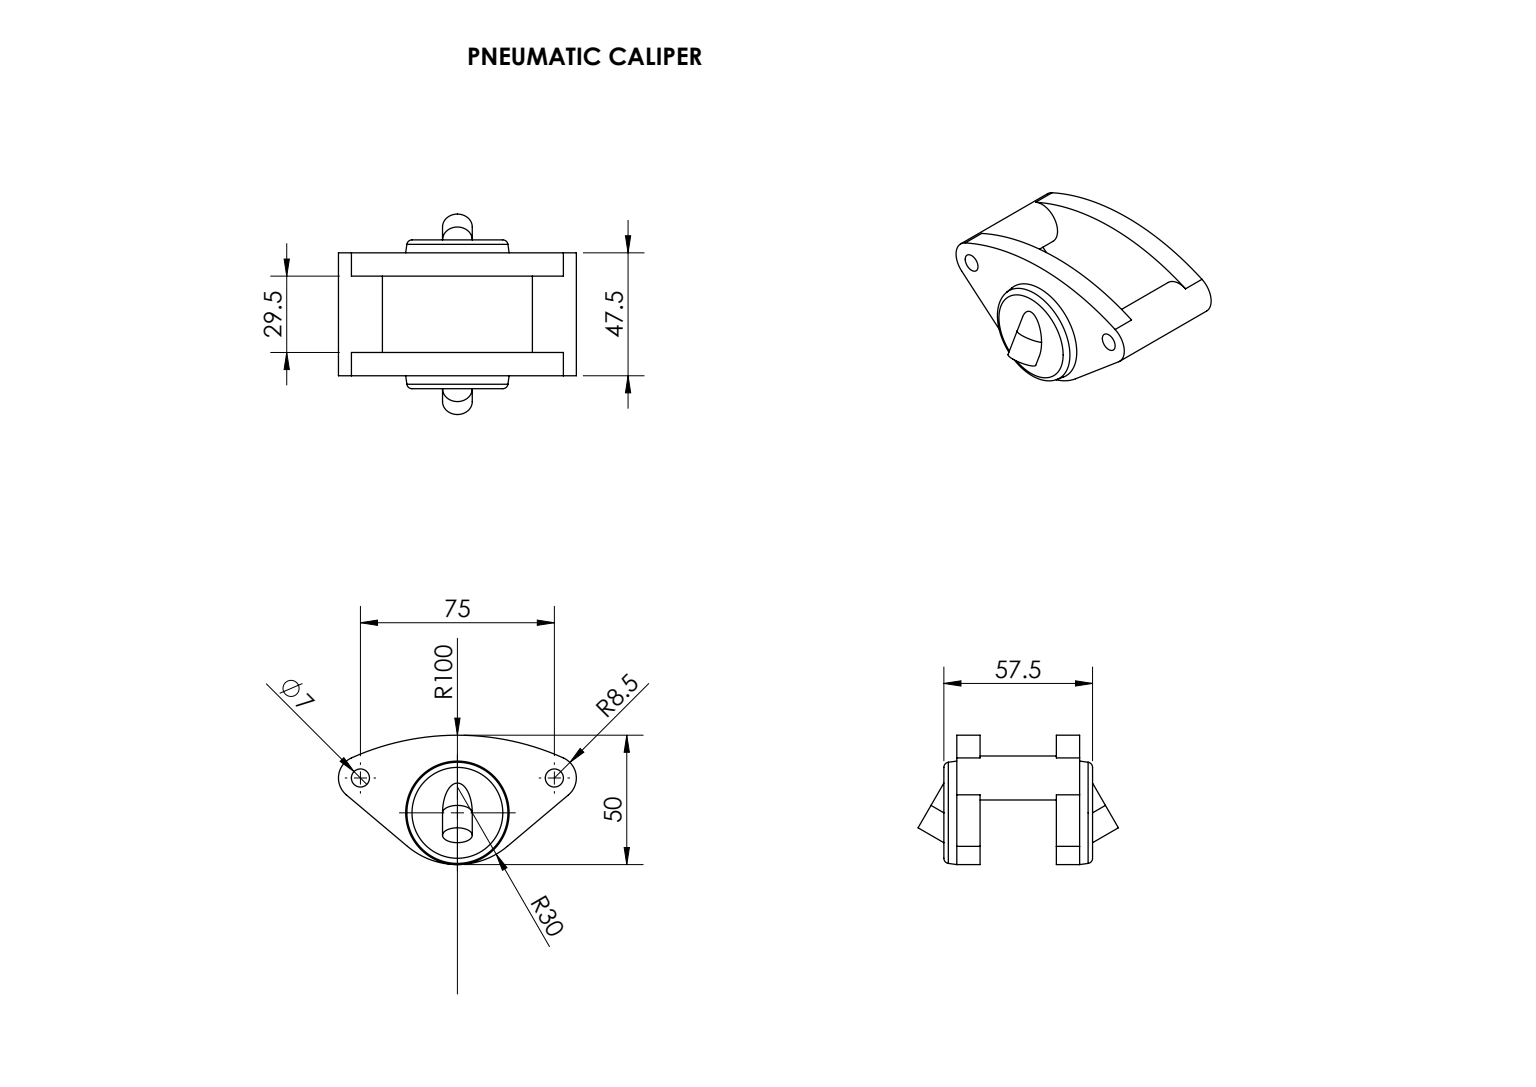
ISO-10303-21;
HEADER;
FILE_DESCRIPTION (('STEP AP214'),
    '1' );
FILE_NAME ('Pneumatic caliper.step',
    '2026-09-21T15:58:29',
    ( '' ),
    ( '' ),
    'SwSTEP 2.0',
    'SolidWorks 2026',
    '' );
FILE_SCHEMA (( 'AUTOMOTIVE_DESIGN' ));
ENDSEC;

DATA;
#6=AXIS2_PLACEMENT_3D ( 'NONE', #11763, #3538, #9529 ) ;
#8=ADVANCED_FACE ( 'NONE', ( #25357 ), #3421, .T. ) ;
#26=DIRECTION ( 'NONE',  ( 0.000000000000000000, 0.4999999999999951150, -0.8660254037844414832 ) ) ;
#43=LINE ( 'NONE', #5489, #22981 ) ;
#65=LINE ( 'NONE', #14323, #21127 ) ;
#74=CARTESIAN_POINT ( 'NONE',  ( -5.750000000000000000, 96.68456697298042002, 32.49999999999999289 ) ) ;
#105=VERTEX_POINT ( 'NONE', #9030 ) ;
#134=ORIENTED_EDGE ( 'NONE', *, *, #2252, .T. ) ;
#160=PRODUCT ( 'Pneumatic caliper', 'Pneumatic caliper', '', ( #18111 ) ) ;
#162=CARTESIAN_POINT ( 'NONE',  ( -2.448772250512182280E-15, 99.94802294027086020, -19.99999999999999645 ) ) ;
#175=CARTESIAN_POINT ( 'NONE',  ( -37.50000000000000000, 103.4105893997321886, -19.99999999999999645 ) ) ;
#283=ORIENTED_EDGE ( 'NONE', *, *, #11463, .F. ) ;
#335=ORIENTED_EDGE ( 'NONE', *, *, #20881, .T. ) ;
#374=VERTEX_POINT ( 'NONE', #8609 ) ;
#431=DIRECTION ( 'NONE',  ( 1.000000000000000000, 0.000000000000000000, 0.000000000000000000 ) ) ;
#441=ORIENTED_EDGE ( 'NONE', *, *, #21012, .F. ) ;
#469=EDGE_CURVE ( 'NONE', #105, #36472, #11048, .T. ) ;
#493=EDGE_CURVE ( 'NONE', #20027, #19694, #7016, .T. ) ;
#530=VERTEX_POINT ( 'NONE', #7444 ) ;
#537=CARTESIAN_POINT ( 'NONE',  ( -37.50000000000000000, 103.4105893997321886, 27.49999999999999645 ) ) ;
#544=CARTESIAN_POINT ( 'NONE',  ( 40.98360655737705116, 111.1639425680974398, -19.99999999999999645 ) ) ;
#554=EDGE_CURVE ( 'NONE', #14180, #7296, #6835, .T. ) ;
#576=CARTESIAN_POINT ( 'NONE',  ( 3.368272016354729725, 78.44802294027070388, 32.49999999999999289 ) ) ;
#585=DIRECTION ( 'NONE',  ( 0.000000000000000000, -0.000000000000000000, 1.000000000000000000 ) ) ;
#623=VERTEX_POINT ( 'NONE', #30682 ) ;
#651=DIRECTION ( 'NONE',  ( 1.000000000000000000, 0.000000000000000000, 0.000000000000000000 ) ) ;
#681=EDGE_CURVE ( 'NONE', #4131, #30183, #32146, .T. ) ;
#692=CYLINDRICAL_SURFACE ( 'NONE', #6427, 5.750000000000005329 ) ;
#705=FACE_OUTER_BOUND ( 'NONE', #31997, .T. ) ;
#721=CARTESIAN_POINT ( 'NONE',  ( 40.98360655737705116, 111.1639425680974398, 27.49999999999999645 ) ) ;
#750=CARTESIAN_POINT ( 'NONE',  ( -7.041719095097282852E-16, 78.44802294027068967, 32.49999999999999289 ) ) ;
#755=VERTEX_POINT ( 'NONE', #25262 ) ;
#856=CARTESIAN_POINT ( 'NONE',  ( 19.31922176934805435, 76.99660315353983719, -11.00000000000000000 ) ) ;
#927=CARTESIAN_POINT ( 'NONE',  ( 46.00000000000000000, 103.4105893997321743, -19.99999999999999645 ) ) ;
#950=EDGE_CURVE ( 'NONE', #15883, #26378, #23725, .T. ) ;
#958=VECTOR ( 'NONE', #35917, 1000.000000000000000 ) ;
#983=AXIS2_PLACEMENT_3D ( 'NONE', #1559, #4573, #18819 ) ;
#1027=CARTESIAN_POINT ( 'NONE',  ( -33.99999999999999289, 103.4105893997321886, -19.99999999999999645 ) ) ;
#1082=CARTESIAN_POINT ( 'NONE',  ( 37.50000000000000000, 103.4105893997321743, -19.99999999999999645 ) ) ;
#1097=DIRECTION ( 'NONE',  ( 0.000000000000000000, -0.8660254037844420383, -0.4999999999999945599 ) ) ;
#1190=ORIENTED_EDGE ( 'NONE', *, *, #24796, .T. ) ;
#1228=ORIENTED_EDGE ( 'NONE', *, *, #33762, .F. ) ;
#1243=DIRECTION ( 'NONE',  ( -0.000000000000000000, -0.000000000000000000, 1.000000000000000000 ) ) ;
#1432=ORIENTED_EDGE ( 'NONE', *, *, #33576, .T. ) ;
#1488=CIRCLE ( 'NONE', #28409, 1.750000000000018652 ) ;
#1509=ORIENTED_EDGE ( 'NONE', *, *, #29374, .F. ) ;
#1513=DIRECTION ( 'NONE',  ( 0.000000000000000000, 0.4999999999999953926, 0.8660254037844412611 ) ) ;
#1518=DIRECTION ( 'NONE',  ( -0.000000000000000000, -0.000000000000000000, 1.000000000000000000 ) ) ;
#1531=ORIENTED_EDGE ( 'NONE', *, *, #950, .F. ) ;
#1540=AXIS2_PLACEMENT_3D ( 'NONE', #7269, #15702, #21694 ) ;
#1559=CARTESIAN_POINT ( 'NONE',  ( 0.000000000000000000, 89.94802294027088863, 27.49999999999999645 ) ) ;
#1579=CARTESIAN_POINT ( 'NONE',  ( 42.97377950131527058, 96.90768712682506703, -19.99999999999999645 ) ) ;
#1619=DIRECTION ( 'NONE',  ( 0.000000000000000000, -0.000000000000000000, 1.000000000000000000 ) ) ;
#1622=EDGE_CURVE ( 'NONE', #20027, #10852, #65, .T. ) ;
#1690=LINE ( 'NONE', #32433, #24985 ) ;
#1707=DIRECTION ( 'NONE',  ( 0.000000000000000000, 0.000000000000000000, 1.000000000000000000 ) ) ;
#1771=CARTESIAN_POINT ( 'NONE',  ( 0.000000000000000000, 84.16276890242652087, 42.47964607176039209 ) ) ;
#1854=ADVANCED_BREP_SHAPE_REPRESENTATION ( '', ( #32508, #21385 ), #29775 ) ;
#1871=PLANE ( 'NONE',  #17245 ) ;
#1872=ORIENTED_EDGE ( 'NONE', *, *, #18822, .T. ) ;
#1907=FACE_BOUND ( 'NONE', #19435, .T. ) ;
#1911=CARTESIAN_POINT ( 'NONE',  ( 0.000000000000000000, 81.28776890242656350, 37.49999999999985079 ) ) ;
#1925=EDGE_LOOP ( 'NONE', ( #10034, #14549, #26368, #1432 ) ) ;
#1928=CARTESIAN_POINT ( 'NONE',  ( 19.31922176934805435, 76.99660315353983719, 18.49999999999999645 ) ) ;
#1999=CARTESIAN_POINT ( 'NONE',  ( 5.750000000000000000, 89.94802294027094547, -24.99999999999999645 ) ) ;
#2018=DIRECTION ( 'NONE',  ( 0.000000000000000000, -0.8660254037844420383, -0.4999999999999945599 ) ) ;
#2092=ADVANCED_FACE ( 'NONE', ( #33123 ), #7443, .F. ) ;
#2180=CARTESIAN_POINT ( 'NONE',  ( -2.775557561562891351E-14, 19.94802294027085310, 27.49999999999999645 ) ) ;
#2187=DIRECTION ( 'NONE',  ( -1.000000000000000000, 0.000000000000000000, 0.000000000000000000 ) ) ;
#2193=CARTESIAN_POINT ( 'NONE',  ( -3.368272016354703968, 101.4480229402710592, 32.49999999999999289 ) ) ;
#2207=ADVANCED_FACE ( 'NONE', ( #24326 ), #10261, .F. ) ;
#2222=AXIS2_PLACEMENT_3D ( 'NONE', #29319, #32113, #20494 ) ;
#2228=ORIENTED_EDGE ( 'NONE', *, *, #950, .T. ) ;
#2252=EDGE_CURVE ( 'NONE', #24938, #36272, #5855, .T. ) ;
#2262=DIRECTION ( 'NONE',  ( -1.000000000000000000, 0.000000000000000000, 0.000000000000000000 ) ) ;
#2268=AXIS2_PLACEMENT_3D ( 'NONE', #6413, #29284, #22929 ) ;
#2294=EDGE_CURVE ( 'NONE', #12700, #36472, #17833, .T. ) ;
#2349=EDGE_CURVE ( 'NONE', #5579, #28337, #19633, .T. ) ;
#2398=AXIS2_PLACEMENT_3D ( 'NONE', #17153, #19603, #14518 ) ;
#2405=AXIS2_PLACEMENT_3D ( 'NONE', #24464, #16022, #21641 ) ;
#2437=FACE_BOUND ( 'NONE', #33052, .T. ) ;
#2439=CYLINDRICAL_SURFACE ( 'NONE', #3558, 5.750000000000002665 ) ;
#2454=CARTESIAN_POINT ( 'NONE',  ( -7.041719095097282852E-16, 87.07302294027100231, 27.52035392823936633 ) ) ;
#2478=DIRECTION ( 'NONE',  ( -0.000000000000000000, -0.000000000000000000, 1.000000000000000000 ) ) ;
#2492=DIRECTION ( 'NONE',  ( -0.000000000000000000, 0.8660254037844420383, -0.4999999999999945599 ) ) ;
#2516=LINE ( 'NONE', #31197, #12942 ) ;
#2582=CYLINDRICAL_SURFACE ( 'NONE', #11940, 8.500000000000003553 ) ;
#2620=CARTESIAN_POINT ( 'NONE',  ( 0.000000000000000000, 89.94802294027088863, 30.77834620192012594 ) ) ;
#2678=DIRECTION ( 'NONE',  ( 0.000000000000000000, 0.000000000000000000, -1.000000000000000000 ) ) ;
#2688=DIRECTION ( 'NONE',  ( -0.000000000000000000, -0.000000000000000000, -1.000000000000000000 ) ) ;
#2707=AXIS2_PLACEMENT_3D ( 'NONE', #5216, #2018, #20008 ) ;
#2814=ORIENTED_EDGE ( 'NONE', *, *, #21581, .T. ) ;
#2937=ORIENTED_EDGE ( 'NONE', *, *, #18375, .T. ) ;
#2945=EDGE_CURVE ( 'NONE', #374, #33065, #32532, .T. ) ;
#2967=DIRECTION ( 'NONE',  ( 0.000000000000000000, 0.000000000000000000, -1.000000000000000000 ) ) ;
#3005=SURFACE_STYLE_USAGE ( .BOTH. , #36939 ) ;
#3025=DIRECTION ( 'NONE',  ( 0.000000000000000000, -0.8660254037844419273, 0.4999999999999945599 ) ) ;
#3049=FACE_BOUND ( 'NONE', #20436, .T. ) ;
#3106=DIRECTION ( 'NONE',  ( -1.000000000000000000, 0.000000000000000000, 0.000000000000000000 ) ) ;
#3130=CARTESIAN_POINT ( 'NONE',  ( 0.000000000000000000, 81.28776890242656350, -29.99999999999985434 ) ) ;
#3139=CARTESIAN_POINT ( 'NONE',  ( 0.000000000000000000, 89.94802294027097389, -24.99999999999990763 ) ) ;
#3154=EDGE_LOOP ( 'NONE', ( #27426, #3715 ) ) ;
#3161=CARTESIAN_POINT ( 'NONE',  ( 0.000000000000000000, 89.94802294027088863, -24.99999999999999645 ) ) ;
#3167=VERTEX_POINT ( 'NONE', #4549 ) ;
#3178=ORIENTED_EDGE ( 'NONE', *, *, #493, .T. ) ;
#3242=LINE ( 'NONE', #17667, #10545 ) ;
#3254=VERTEX_POINT ( 'NONE', #22529 ) ;
#3267=DIRECTION ( 'NONE',  ( 1.000000000000000000, 0.000000000000000000, 0.000000000000000000 ) ) ;
#3338=ORIENTED_EDGE ( 'NONE', *, *, #7196, .T. ) ;
#3362=VECTOR ( 'NONE', #20623, 1000.000000000000000 ) ;
#3404=ORIENTED_EDGE ( 'NONE', *, *, #19687, .T. ) ;
#3411=DIRECTION ( 'NONE',  ( 0.000000000000000000, -1.000000000000000000, 0.000000000000000000 ) ) ;
#3415=AXIS2_PLACEMENT_3D ( 'NONE', #24206, #30396, #7341 ) ;
#3421=TOROIDAL_SURFACE ( 'NONE', #24386, 17.55872235085560007, 2.000000000000000000 ) ;
#3425=CARTESIAN_POINT ( 'NONE',  ( 37.50000000000000000, 103.4105893997321743, -19.99999999999999645 ) ) ;
#3432=VERTEX_POINT ( 'NONE', #34894 ) ;
#3476=AXIS2_PLACEMENT_3D ( 'NONE', #10985, #5195, #16826 ) ;
#3492=ORIENTED_EDGE ( 'NONE', *, *, #17442, .F. ) ;
#3538=DIRECTION ( 'NONE',  ( -0.000000000000000000, -0.000000000000000000, 1.000000000000000000 ) ) ;
#3550=ORIENTED_EDGE ( 'NONE', *, *, #19687, .F. ) ;
#3558=AXIS2_PLACEMENT_3D ( 'NONE', #31282, #17035, #28469 ) ;
#3585=CARTESIAN_POINT ( 'NONE',  ( 5.750000000000035527, 83.21147890756138565, 32.49999999999999289 ) ) ;
#3645=LINE ( 'NONE', #15074, #20651 ) ;
#3651=CARTESIAN_POINT ( 'NONE',  ( -28.99999999999998934, 103.4105893997321886, -11.00000000000000355 ) ) ;
#3715=ORIENTED_EDGE ( 'NONE', *, *, #27481, .F. ) ;
#3739=DIRECTION ( 'NONE',  ( 1.000000000000000000, 0.000000000000000000, 0.000000000000000000 ) ) ;
#3743=FACE_OUTER_BOUND ( 'NONE', #7188, .T. ) ;
#3776=DIRECTION ( 'NONE',  ( -0.000000000000000000, -0.000000000000000000, 1.000000000000000000 ) ) ;
#3779=DIRECTION ( 'NONE',  ( 0.000000000000000000, 0.000000000000000000, -1.000000000000000000 ) ) ;
#3785=DIRECTION ( 'NONE',  ( -1.000000000000000000, 0.000000000000000000, 0.000000000000000000 ) ) ;
#3796=ORIENTED_EDGE ( 'NONE', *, *, #31417, .F. ) ;
#3819=ADVANCED_FACE ( 'NONE', ( #28664 ), #2439, .T. ) ;
#3840=DIRECTION ( 'NONE',  ( -0.000000000000000000, -0.000000000000000000, -1.000000000000000000 ) ) ;
#3868=CARTESIAN_POINT ( 'NONE',  ( 0.000000000000000000, 98.60827697811544112, -19.99999999999999645 ) ) ;
#3871=VECTOR ( 'NONE', #23270, 1000.000000000000000 ) ;
#3883=DIRECTION ( 'NONE',  ( 0.6439740589782694258, 0.7650473262243666639, 0.000000000000000000 ) ) ;
#3895=CIRCLE ( 'NONE', #24270, 17.55872235085560007 ) ;
#3909=ORIENTED_EDGE ( 'NONE', *, *, #33038, .T. ) ;
#3956=VECTOR ( 'NONE', #20517, 1000.000000000000000 ) ;
#3970=LINE ( 'NONE', #6607, #19644 ) ;
#3978=CARTESIAN_POINT ( 'NONE',  ( 37.50000000000000000, 103.4105893997321743, -11.00000000000000355 ) ) ;
#3980=CARTESIAN_POINT ( 'NONE',  ( -42.97377950131527058, 96.90768712682508124, 18.49999999999999645 ) ) ;
#4025=CARTESIAN_POINT ( 'NONE',  ( -28.99999999999998934, 103.4105893997321886, 18.49999999999999645 ) ) ;
#4050=VERTEX_POINT ( 'NONE', #5357 ) ;
#4058=EDGE_CURVE ( 'NONE', #16958, #13946, #30472, .T. ) ;
#4094=FILL_AREA_STYLE_COLOUR ( '', #11095 ) ;
#4096=AXIS2_PLACEMENT_3D ( 'NONE', #31153, #25722, #11273 ) ;
#4099=DIRECTION ( 'NONE',  ( -0.000000000000000000, -0.000000000000000000, -1.000000000000000000 ) ) ;
#4131=VERTEX_POINT ( 'NONE', #30645 ) ;
#4151=CARTESIAN_POINT ( 'NONE',  ( 19.31922176934805435, 76.99660315353983719, -19.99999999999999645 ) ) ;
#4153=VECTOR ( 'NONE', #5154, 1000.000000000000000 ) ;
#4164=ORIENTED_EDGE ( 'NONE', *, *, #15491, .F. ) ;
#4167=ORIENTED_EDGE ( 'NONE', *, *, #23423, .F. ) ;
#4229=DIRECTION ( 'NONE',  ( -0.000000000000000000, -0.000000000000000000, -1.000000000000000000 ) ) ;
#4230=ORIENTED_EDGE ( 'NONE', *, *, #10722, .F. ) ;
#4234=EDGE_LOOP ( 'NONE', ( #22115, #32877 ) ) ;
#4257=CARTESIAN_POINT ( 'NONE',  ( 0.000000000000000000, 85.61789592134881843, -27.49999999999990408 ) ) ;
#4343=CARTESIAN_POINT ( 'NONE',  ( 0.000000000000000000, 98.60827697811544112, 27.49999999999999645 ) ) ;
#4363=ORIENTED_EDGE ( 'NONE', *, *, #23423, .T. ) ;
#4408=AXIS2_PLACEMENT_3D ( 'NONE', #21823, #33261, #16774 ) ;
#4410=CARTESIAN_POINT ( 'NONE',  ( 37.50000000000000000, 103.4105893997321743, 27.49999999999999645 ) ) ;
#4445=AXIS2_PLACEMENT_3D ( 'NONE', #30967, #8096, #25528 ) ;
#4450=DIRECTION ( 'NONE',  ( -0.000000000000000000, -0.000000000000000000, -1.000000000000000000 ) ) ;
#4475=ORIENTED_EDGE ( 'NONE', *, *, #30097, .T. ) ;
#4479=VECTOR ( 'NONE', #26592, 1000.000000000000000 ) ;
#4530=DIRECTION ( 'NONE',  ( -0.000000000000000000, -0.8660254037844414832, 0.4999999999999953371 ) ) ;
#4549=CARTESIAN_POINT ( 'NONE',  ( 7.041719095097282852E-16, 78.41276890242659192, -25.02035392823930593 ) ) ;
#4556=VERTEX_POINT ( 'NONE', #4560 ) ;
#4560=CARTESIAN_POINT ( 'NONE',  ( -7.041719095097282852E-16, 78.44802294027068967, 32.49999999999999289 ) ) ;
#4571=ORIENTED_EDGE ( 'NONE', *, *, #11658, .F. ) ;
#4573=DIRECTION ( 'NONE',  ( 0.000000000000000000, 0.000000000000000000, -1.000000000000000000 ) ) ;
#4580=FACE_BOUND ( 'NONE', #4234, .T. ) ;
#4585=LINE ( 'NONE', #24827, #34492 ) ;
#4596=EDGE_CURVE ( 'NONE', #34855, #18201, #32666, .T. ) ;
#4610=VERTEX_POINT ( 'NONE', #20447 ) ;
#4626=ADVANCED_FACE ( 'NONE', ( #28524, #28718, #3049 ), #28332, .F. ) ;
#4627=CARTESIAN_POINT ( 'NONE',  ( 0.000000000000000000, 82.16276890242660613, -31.51554445662266346 ) ) ;
#4633=CARTESIAN_POINT ( 'NONE',  ( 0.000000000000000000, 81.28776890242660613, -29.99999999999987566 ) ) ;
#4651=ORIENTED_EDGE ( 'NONE', *, *, #21027, .F. ) ;
#4666=CIRCLE ( 'NONE', #24411, 20.00000000000001066 ) ;
#4734=ORIENTED_EDGE ( 'NONE', *, *, #30255, .T. ) ;
#4760=VERTEX_POINT ( 'NONE', #35081 ) ;
#4769=AXIS2_PLACEMENT_3D ( 'NONE', #27991, #7760, #16371 ) ;
#4812=ORIENTED_EDGE ( 'NONE', *, *, #35492, .T. ) ;
#4827=EDGE_CURVE ( 'NONE', #22247, #15238, #15196, .T. ) ;
#4922=ORIENTED_EDGE ( 'NONE', *, *, #23505, .T. ) ;
#4934=DIRECTION ( 'NONE',  ( 0.000000000000000000, -0.8660254037844419273, 0.4999999999999945044 ) ) ;
#4964=CARTESIAN_POINT ( 'NONE',  ( 0.000000000000000000, 89.94802294027088863, 27.49999999999999645 ) ) ;
#5066=CARTESIAN_POINT ( 'NONE',  ( -41.00000000000000000, 103.4105893997321886, -19.99999999999999645 ) ) ;
#5149=ORIENTED_EDGE ( 'NONE', *, *, #31933, .T. ) ;
#5154=DIRECTION ( 'NONE',  ( -0.7650473262243666639, 0.6439740589782693148, -0.000000000000000000 ) ) ;
#5164=VECTOR ( 'NONE', #15215, 1000.000000000000114 ) ;
#5181=ADVANCED_FACE ( 'NONE', ( #32325 ), #28520, .T. ) ;
#5195=DIRECTION ( 'NONE',  ( -0.000000000000000000, -0.000000000000000000, -1.000000000000000000 ) ) ;
#5206=CARTESIAN_POINT ( 'NONE',  ( 0.000000000000000000, 101.4480229402710592, -24.99999999999999645 ) ) ;
#5216=CARTESIAN_POINT ( 'NONE',  ( 0.000000000000000000, 81.28776890242656350, -29.99999999999985434 ) ) ;
#5217=AXIS2_PLACEMENT_3D ( 'NONE', #21560, #24571, #32991 ) ;
#5218=FACE_OUTER_BOUND ( 'NONE', #16123, .T. ) ;
#5245=CIRCLE ( 'NONE', #6439, 8.500000000000000000 ) ;
#5256=STYLED_ITEM ( 'NONE', ( #28128 ), #1854 ) ;
#5266=FILL_AREA_STYLE ('',( #5811 ) ) ;
#5300=CIRCLE ( 'NONE', #30417, 2.000000000000001776 ) ;
#5329=ORIENTED_EDGE ( 'NONE', *, *, #24410, .F. ) ;
#5357=CARTESIAN_POINT ( 'NONE',  ( 40.98360655737705827, 111.1639425680974540, -11.00000000000000355 ) ) ;
#5428=CARTESIAN_POINT ( 'NONE',  ( 0.000000000000000000, 89.94802294027088863, 27.49999999999999645 ) ) ;
#5448=ADVANCED_FACE ( 'NONE', ( #20294 ), #31526, .F. ) ;
#5489=CARTESIAN_POINT ( 'NONE',  ( 0.000000000000000000, 86.49289592134881843, -29.01554445662268833 ) ) ;
#5512=CARTESIAN_POINT ( 'NONE',  ( 42.97377950131527058, 96.90768712682506703, -11.00000000000000000 ) ) ;
#5577=CARTESIAN_POINT ( 'NONE',  ( 0.000000000000000000, 89.94802294027094547, 32.49999999999999289 ) ) ;
#5579=VERTEX_POINT ( 'NONE', #13277 ) ;
#5591=FACE_OUTER_BOUND ( 'NONE', #29113, .T. ) ;
#5613=( NAMED_UNIT ( * ) PLANE_ANGLE_UNIT ( ) SI_UNIT ( $, .RADIAN. ) );
#5627=DIRECTION ( 'NONE',  ( 0.000000000000000000, -0.8660254037844419273, -0.4999999999999945599 ) ) ;
#5649=CIRCLE ( 'NONE', #35593, 19.53925848833874213 ) ;
#5652=VECTOR ( 'NONE', #24376, 1000.000000000000000 ) ;
#5665=CARTESIAN_POINT ( 'NONE',  ( 0.000000000000000000, 81.28776890242656350, 37.49999999999985079 ) ) ;
#5710=AXIS2_PLACEMENT_3D ( 'NONE', #29491, #23899, #34952 ) ;
#5712=CYLINDRICAL_SURFACE ( 'NONE', #27964, 5.750000000000002665 ) ;
#5755=CIRCLE ( 'NONE', #10513, 8.500000000000003553 ) ;
#5768=DIRECTION ( 'NONE',  ( -0.000000000000000000, -0.000000000000000000, 1.000000000000000000 ) ) ;
#5782=CIRCLE ( 'NONE', #10573, 5.750000000000005329 ) ;
#5811=FILL_AREA_STYLE_COLOUR ( '', #29097 ) ;
#5832=CARTESIAN_POINT ( 'NONE',  ( -2.775557561562891351E-14, 19.94802294027085310, 18.49999999999999645 ) ) ;
#5849=ORIENTED_EDGE ( 'NONE', *, *, #21287, .T. ) ;
#5852=CARTESIAN_POINT ( 'NONE',  ( 41.00000000000000000, 103.4105893997321743, -19.99999999999999645 ) ) ;
#5853=DIRECTION ( 'NONE',  ( 1.000000000000000000, 0.000000000000000000, 0.000000000000000000 ) ) ;
#5855=CIRCLE ( 'NONE', #8268, 1.750000000000015765 ) ;
#5892=VECTOR ( 'NONE', #6515, 999.9999999999998863 ) ;
#5900=ORIENTED_EDGE ( 'NONE', *, *, #31535, .F. ) ;
#5904=ADVANCED_FACE ( 'NONE', ( #31800 ), #692, .T. ) ;
#5941=EDGE_LOOP ( 'NONE', ( #16432, #3338, #5149, #21200 ) ) ;
#5956=DIRECTION ( 'NONE',  ( -0.000000000000000000, 0.000000000000000000, -1.000000000000000000 ) ) ;
#5970=CYLINDRICAL_SURFACE ( 'NONE', #29208, 5.750000000000002665 ) ;
#5977=AXIS2_PLACEMENT_3D ( 'NONE', #8755, #5956, #17387 ) ;
#6063=CARTESIAN_POINT ( 'NONE',  ( -2.448772250512182280E-15, 99.94802294027086020, 18.49999999999999645 ) ) ;
#6143=DIRECTION ( 'NONE',  ( -1.000000000000000000, 1.632680918566405215E-15, 0.000000000000000000 ) ) ;
#6151=EDGE_CURVE ( 'NONE', #16958, #30923, #25075, .T. ) ;
#6179=LINE ( 'NONE', #8815, #21940 ) ;
#6216=LINE ( 'NONE', #17648, #15504 ) ;
#6225=AXIS2_PLACEMENT_3D ( 'NONE', #4410, #3840, #29708 ) ;
#6236=ORIENTED_EDGE ( 'NONE', *, *, #10351, .T. ) ;
#6252=VERTEX_POINT ( 'NONE', #22808 ) ;
#6253=VERTEX_POINT ( 'NONE', #8543 ) ;
#6258=ORIENTED_EDGE ( 'NONE', *, *, #31855, .F. ) ;
#6299=DIRECTION ( 'NONE',  ( 0.000000000000000000, -0.8660254037844420383, -0.4999999999999945599 ) ) ;
#6312=DIRECTION ( 'NONE',  ( 0.000000000000000000, 0.4999999999999953926, -0.8660254037844412611 ) ) ;
#6384=CARTESIAN_POINT ( 'NONE',  ( -5.750000000000000000, 89.94802294027094547, -24.99999999999999645 ) ) ;
#6413=CARTESIAN_POINT ( 'NONE',  ( 37.50000000000000000, 103.4105893997321743, 27.49999999999999645 ) ) ;
#6422=DIRECTION ( 'NONE',  ( -0.000000000000000000, -0.000000000000000000, -1.000000000000000000 ) ) ;
#6427=AXIS2_PLACEMENT_3D ( 'NONE', #3139, #6514, #12493 ) ;
#6439=AXIS2_PLACEMENT_3D ( 'NONE', #19759, #30451, #7942 ) ;
#6480=CIRCLE ( 'NONE', #14876, 5.750000000000002665 ) ;
#6481=CARTESIAN_POINT ( 'NONE',  ( 37.50000000000000000, 103.4105893997321743, -19.99999999999999645 ) ) ;
#6490=CARTESIAN_POINT ( 'NONE',  ( -5.750000000000000000, 89.94802294027094547, -24.99999999999999645 ) ) ;
#6514=DIRECTION ( 'NONE',  ( 0.000000000000000000, -0.8660254037844419273, -0.4999999999999945599 ) ) ;
#6515=DIRECTION ( 'NONE',  ( 0.1391731009600657432, 1.704378926181559679E-17, -0.9902680687415703620 ) ) ;
#6533=VERTEX_POINT ( 'NONE', #35527 ) ;
#6576=ADVANCED_FACE ( 'NONE', ( #4580, #30066 ), #35367, .T. ) ;
#6607=CARTESIAN_POINT ( 'NONE',  ( 42.97377950131527058, 96.90768712682506703, -19.99999999999999645 ) ) ;
#6618=DIRECTION ( 'NONE',  ( -0.7650473262243666639, 0.6439740589782693148, 0.000000000000000000 ) ) ;
#6691=ORIENTED_EDGE ( 'NONE', *, *, #30948, .F. ) ;
#6710=EDGE_CURVE ( 'NONE', #6874, #5579, #15562, .T. ) ;
#6753=CARTESIAN_POINT ( 'NONE',  ( -5.750000000000000000, 96.68456697298042002, -25.00000000000000000 ) ) ;
#6815=CIRCLE ( 'NONE', #8027, 8.500000000000007105 ) ;
#6819=VERTEX_POINT ( 'NONE', #13710 ) ;
#6835=( BOUNDED_CURVE ( )  B_SPLINE_CURVE ( 3, ( #21877, #16092, #24328, #1999 ),
 .UNSPECIFIED., .F., .F. ) 
 B_SPLINE_CURVE_WITH_KNOTS ( ( 4, 4 ),
 ( 3.141592653589793116, 4.712388980384689674 ),
 .UNSPECIFIED. ) 
 CURVE ( )  GEOMETRIC_REPRESENTATION_ITEM ( )  RATIONAL_B_SPLINE_CURVE ( ( 1.000000000000000000, 0.8047378541243649375, 0.8047378541243649375, 1.000000000000000000 ) ) 
 REPRESENTATION_ITEM ( '' )  );
#6841=CIRCLE ( 'NONE', #11616, 8.500000000000007105 ) ;
#6874=VERTEX_POINT ( 'NONE', #31839 ) ;
#6885=ORIENTED_EDGE ( 'NONE', *, *, #26374, .T. ) ;
#6923=DIRECTION ( 'NONE',  ( -0.000000000000000000, -0.000000000000000000, 1.000000000000000000 ) ) ;
#6925=AXIS2_PLACEMENT_3D ( 'NONE', #1082, #21519, #32566 ) ;
#6928=ORIENTED_EDGE ( 'NONE', *, *, #4058, .F. ) ;
#6933=CARTESIAN_POINT ( 'NONE',  ( 5.750000000000000000, 89.94802294027094547, -24.99999999999999645 ) ) ;
#6938=EDGE_LOOP ( 'NONE', ( #4475, #19535, #15637, #7352 ) ) ;
#6982=ORIENTED_EDGE ( 'NONE', *, *, #554, .F. ) ;
#7000=ORIENTED_EDGE ( 'NONE', *, *, #14837, .F. ) ;
#7016=CIRCLE ( 'NONE', #31542, 30.00000000000001421 ) ;
#7172=CARTESIAN_POINT ( 'NONE',  ( 7.041719095097282852E-16, 87.07302294027100231, -20.02035392823936633 ) ) ;
#7188=EDGE_LOOP ( 'NONE', ( #25721, #32984, #36736, #7326, #1228 ) ) ;
#7196=EDGE_CURVE ( 'NONE', #6819, #9156, #26992, .T. ) ;
#7223=DIRECTION ( 'NONE',  ( -0.6439740589782688707, 0.7650473262243671080, 0.000000000000000000 ) ) ;
#7269=CARTESIAN_POINT ( 'NONE',  ( -37.50000000000000000, 103.4105893997321886, -19.99999999999999645 ) ) ;
#7275=DIRECTION ( 'NONE',  ( 0.000000000000000000, 0.000000000000000000, 1.000000000000000000 ) ) ;
#7296=VERTEX_POINT ( 'NONE', #32339 ) ;
#7312=DIRECTION ( 'NONE',  ( -0.000000000000000000, -0.000000000000000000, 1.000000000000000000 ) ) ;
#7319=CARTESIAN_POINT ( 'NONE',  ( 40.98360655737705116, 111.1639425680974398, 18.49999999999999645 ) ) ;
#7324=EDGE_CURVE ( 'NONE', #4760, #12700, #11711, .T. ) ;
#7326=ORIENTED_EDGE ( 'NONE', *, *, #29029, .F. ) ;
#7341=DIRECTION ( 'NONE',  ( -1.000000000000000000, 0.000000000000000000, 0.000000000000000000 ) ) ;
#7352=ORIENTED_EDGE ( 'NONE', *, *, #32835, .T. ) ;
#7405=EDGE_LOOP ( 'NONE', ( #22340, #26272, #16422, #30979, #30208, #12182, #13169, #4363 ) ) ;
#7432=CARTESIAN_POINT ( 'NONE',  ( -37.50000000000000000, 103.4105893997321743, -11.00000000000000355 ) ) ;
#7443=CYLINDRICAL_SURFACE ( 'NONE', #6925, 3.500000000000003109 ) ;
#7444=CARTESIAN_POINT ( 'NONE',  ( 33.99999999999999289, 103.4105893997321743, 27.49999999999999645 ) ) ;
#7476=ORIENTED_EDGE ( 'NONE', *, *, #23774, .T. ) ;
#7526=LINE ( 'NONE', #7172, #36324 ) ;
#7576=AXIS2_PLACEMENT_3D ( 'NONE', #21122, #12675, #12496 ) ;
#7624=CIRCLE ( 'NONE', #11288, 8.500000000000007105 ) ;
#7760=DIRECTION ( 'NONE',  ( -0.000000000000000000, -0.000000000000000000, 1.000000000000000000 ) ) ;
#7837=DIRECTION ( 'NONE',  ( 1.000000000000000000, 0.000000000000000000, 0.000000000000000000 ) ) ;
#7856=CONICAL_SURFACE ( 'NONE', #29977, 20.00000000000001066, 0.1396263401595466691 ) ;
#7877=DIRECTION ( 'NONE',  ( -0.000000000000000000, 0.8660254037844420383, -0.4999999999999945599 ) ) ;
#7942=DIRECTION ( 'NONE',  ( -1.000000000000000000, 0.000000000000000000, 0.000000000000000000 ) ) ;
#8005=( NAMED_UNIT ( * ) PLANE_ANGLE_UNIT ( ) SI_UNIT ( $, .RADIAN. ) );
#8027=AXIS2_PLACEMENT_3D ( 'NONE', #29000, #34838, #6143 ) ;
#8049=AXIS2_PLACEMENT_3D ( 'NONE', #26425, #31679, #23252 ) ;
#8062=( LENGTH_UNIT ( ) NAMED_UNIT ( * ) SI_UNIT ( .MILLI., .METRE. ) );
#8071=EDGE_CURVE ( 'NONE', #21230, #13656, #20391, .T. ) ;
#8077=AXIS2_PLACEMENT_3D ( 'NONE', #20063, #3025, #11800 ) ;
#8091=CARTESIAN_POINT ( 'NONE',  ( -37.50000000000000000, 103.4105893997321743, -11.00000000000000355 ) ) ;
#8096=DIRECTION ( 'NONE',  ( -0.6439740589782688707, 0.7650473262243671080, 0.000000000000000000 ) ) ;
#8099=ORIENTED_EDGE ( 'NONE', *, *, #32739, .T. ) ;
#8128=CARTESIAN_POINT ( 'NONE',  ( 37.50000000000000000, 103.4105893997321743, -19.99999999999999645 ) ) ;
#8153=ORIENTED_EDGE ( 'NONE', *, *, #19407, .T. ) ;
#8173=ORIENTED_EDGE ( 'NONE', *, *, #14783, .T. ) ;
#8238=DIRECTION ( 'NONE',  ( -0.000000000000000000, -0.000000000000000000, 1.000000000000000000 ) ) ;
#8268=AXIS2_PLACEMENT_3D ( 'NONE', #29953, #12508, #18529 ) ;
#8288=EDGE_LOOP ( 'NONE', ( #11562, #9328, #11716, #17597 ) ) ;
#8307=CIRCLE ( 'NONE', #23249, 1.750000000000018652 ) ;
#8310=EDGE_LOOP ( 'NONE', ( #4734, #2937, #10628, #15493, #14734, #7476, #21866, #22793, #13839, #3492, #33409, #26878 ) ) ;
#8328=CARTESIAN_POINT ( 'NONE',  ( -37.50000000000000000, 103.4105893997321886, -19.99999999999999645 ) ) ;
#8343=VERTEX_POINT ( 'NONE', #927 ) ;
#8360=EDGE_LOOP ( 'NONE', ( #20679, #10568, #20480, #25399, #35579, #18853, #8988, #28562 ) ) ;
#8402=ADVANCED_FACE ( 'NONE', ( #21922 ), #7856, .T. ) ;
#8444=DIRECTION ( 'NONE',  ( -0.000000000000000000, -0.8660254037844413721, 0.4999999999999952816 ) ) ;
#8461=EDGE_LOOP ( 'NONE', ( #16036, #26770, #33752, #35525 ) ) ;
#8464=VERTEX_POINT ( 'NONE', #27720 ) ;
#8514=ADVANCED_FACE ( 'NONE', ( #5591 ), #31781, .T. ) ;
#8529=CIRCLE ( 'NONE', #28270, 20.00000000000001066 ) ;
#8543=CARTESIAN_POINT ( 'NONE',  ( 0.000000000000000000, 84.16276890242652087, -34.97964607176039920 ) ) ;
#8586=CARTESIAN_POINT ( 'NONE',  ( 0.000000000000000000, 89.94802294027088863, -23.00000000000000000 ) ) ;
#8595=ORIENTED_EDGE ( 'NONE', *, *, #29123, .T. ) ;
#8609=CARTESIAN_POINT ( 'NONE',  ( 17.55872235085560007, 89.94802294027088863, 32.49999999999999289 ) ) ;
#8633=LINE ( 'NONE', #17616, #23182 ) ;
#8645=CARTESIAN_POINT ( 'NONE',  ( -2.448772250512182280E-15, 99.94802294027086020, -11.00000000000000000 ) ) ;
#8755=CARTESIAN_POINT ( 'NONE',  ( -2.775557561562891351E-14, 19.94802294027085310, -11.00000000000000000 ) ) ;
#8760=DIRECTION ( 'NONE',  ( 0.000000000000000000, 0.4999999999999953926, 0.8660254037844412611 ) ) ;
#8797=SHAPE_REPRESENTATION_RELATIONSHIP ( 'NONE' , 'NONE' ,  #35880, #1854 ) ;
#8800=DIRECTION ( 'NONE',  ( -1.000000000000000000, 0.000000000000000000, 0.000000000000000000 ) ) ;
#8814=DIRECTION ( 'NONE',  ( -1.000000000000000000, 0.000000000000000000, 0.000000000000000000 ) ) ;
#8815=CARTESIAN_POINT ( 'NONE',  ( 42.97377950131529190, 96.90768712682505281, 27.49999999999999645 ) ) ;
#8824=CYLINDRICAL_SURFACE ( 'NONE', #4096, 5.750000000000002665 ) ;
#8855=DIRECTION ( 'NONE',  ( 0.000000000000000000, 0.000000000000000000, -1.000000000000000000 ) ) ;
#8862=CARTESIAN_POINT ( 'NONE',  ( 0.000000000000000000, 85.61789592134881843, -27.49999999999990408 ) ) ;
#8882=DIRECTION ( 'NONE',  ( 0.000000000000000000, 0.000000000000000000, 1.000000000000000000 ) ) ;
#8896=CARTESIAN_POINT ( 'NONE',  ( 0.000000000000000000, 0.000000000000000000, 0.000000000000000000 ) ) ;
#8945=EDGE_CURVE ( 'NONE', #15238, #30923, #11687, .T. ) ;
#8954=CIRCLE ( 'NONE', #31118, 5.750000000000002665 ) ;
#8988=ORIENTED_EDGE ( 'NONE', *, *, #15128, .F. ) ;
#9029=VERTEX_POINT ( 'NONE', #32968 ) ;
#9030=CARTESIAN_POINT ( 'NONE',  ( -41.00000000000000000, 103.4105893997321886, -19.99999999999999645 ) ) ;
#9034=EDGE_LOOP ( 'NONE', ( #33361, #6885, #23497, #25388 ) ) ;
#9088=CARTESIAN_POINT ( 'NONE',  ( 0.000000000000000000, 89.94802294027088863, 32.49999999999999289 ) ) ;
#9112=CARTESIAN_POINT ( 'NONE',  ( 4.897544501024384282E-15, 69.94802294027087441, -19.99999999999999645 ) ) ;
#9124=CARTESIAN_POINT ( 'NONE',  ( -19.31922176934808633, 76.99660315353983719, -19.99999999999999645 ) ) ;
#9127=ORIENTED_EDGE ( 'NONE', *, *, #22966, .T. ) ;
#9142=CYLINDRICAL_SURFACE ( 'NONE', #26544, 30.00000000000001421 ) ;
#9148=CIRCLE ( 'NONE', #27115, 3.500000000000003109 ) ;
#9156=VERTEX_POINT ( 'NONE', #33339 ) ;
#9236=( BOUNDED_CURVE ( )  B_SPLINE_CURVE ( 3, ( #31604, #23732, #17924, #6490 ),
 .UNSPECIFIED., .F., .F. ) 
 B_SPLINE_CURVE_WITH_KNOTS ( ( 4, 4 ),
 ( 0.000000000000000000, 1.570796326794907438 ),
 .UNSPECIFIED. ) 
 CURVE ( )  GEOMETRIC_REPRESENTATION_ITEM ( )  RATIONAL_B_SPLINE_CURVE ( ( 1.000000000000000000, 0.8047378541243623840, 0.8047378541243623840, 1.000000000000000000 ) ) 
 REPRESENTATION_ITEM ( '' )  );
#9261=ORIENTED_EDGE ( 'NONE', *, *, #27481, .T. ) ;
#9328=ORIENTED_EDGE ( 'NONE', *, *, #32739, .F. ) ;
#9334=ORIENTED_EDGE ( 'NONE', *, *, #19829, .F. ) ;
#9370=DIRECTION ( 'NONE',  ( 1.000000000000000000, 0.000000000000000000, 0.000000000000000000 ) ) ;
#9468=CARTESIAN_POINT ( 'NONE',  ( -2.775557561562891351E-14, 19.94802294027085310, -19.99999999999999645 ) ) ;
#9483=DIRECTION ( 'NONE',  ( -1.000000000000000000, 0.000000000000000000, 0.000000000000000000 ) ) ;
#9496=CARTESIAN_POINT ( 'NONE',  ( -37.50000000000000000, 103.4105893997321886, -19.99999999999999645 ) ) ;
#9529=DIRECTION ( 'NONE',  ( 1.000000000000000000, 0.000000000000000000, 0.000000000000000000 ) ) ;
#9538=ORIENTED_EDGE ( 'NONE', *, *, #35957, .F. ) ;
#9541=VECTOR ( 'NONE', #15506, 1000.000000000000000 ) ;
#9650=CARTESIAN_POINT ( 'NONE',  ( 0.000000000000000000, 92.82302294027094547, -29.97964607176044893 ) ) ;
#9768=ORIENTED_EDGE ( 'NONE', *, *, #27321, .T. ) ;
#9777=DIRECTION ( 'NONE',  ( 0.000000000000000000, 0.000000000000000000, -1.000000000000000000 ) ) ;
#9807=CYLINDRICAL_SURFACE ( 'NONE', #16668, 100.0000000000000142 ) ;
#9941=UNCERTAINTY_MEASURE_WITH_UNIT (LENGTH_MEASURE( 1.000000000000000082E-05 ), #37074, 'distance_accuracy_value', 'NONE');
#9964=CARTESIAN_POINT ( 'NONE',  ( -19.53925848833874213, 89.94802294027088863, -23.27834620192013304 ) ) ;
#9979=CIRCLE ( 'NONE', #36334, 8.500000000000007105 ) ;
#10022=AXIS2_PLACEMENT_3D ( 'NONE', #27386, #1707, #10317 ) ;
#10034=ORIENTED_EDGE ( 'NONE', *, *, #15128, .T. ) ;
#10035=ORIENTED_EDGE ( 'NONE', *, *, #17199, .T. ) ;
#10065=ADVANCED_FACE ( 'NONE', ( #24398 ), #33990, .T. ) ;
#10082=VECTOR ( 'NONE', #25009, 1000.000000000000000 ) ;
#10092=SURFACE_SIDE_STYLE ('',( #12689 ) ) ;
#10126=FACE_OUTER_BOUND ( 'NONE', #35456, .T. ) ;
#10172=CARTESIAN_POINT ( 'NONE',  ( 0.000000000000000000, 89.94802294027088863, -19.99999999999999645 ) ) ;
#10175=DIRECTION ( 'NONE',  ( -1.000000000000000000, 0.000000000000000000, -0.000000000000000000 ) ) ;
#10199=CARTESIAN_POINT ( 'NONE',  ( -5.750000000000000000, 89.94802294027094547, 32.49999999999999289 ) ) ;
#10245=CARTESIAN_POINT ( 'NONE',  ( 46.00000000000000000, 103.4105893997321743, -19.99999999999999645 ) ) ;
#10261=CYLINDRICAL_SURFACE ( 'NONE', #1540, 3.500000000000003109 ) ;
#10316=CONICAL_SURFACE ( 'NONE', #25289, 20.00000000000001066, 0.1396263401595466691 ) ;
#10317=DIRECTION ( 'NONE',  ( 1.000000000000000000, 0.000000000000000000, 0.000000000000000000 ) ) ;
#10351=EDGE_CURVE ( 'NONE', #623, #4050, #31468, .T. ) ;
#10418=VECTOR ( 'NONE', #24423, 1000.000000000000114 ) ;
#10429=DIRECTION ( 'NONE',  ( -0.000000000000000000, 0.000000000000000000, -1.000000000000000000 ) ) ;
#10485=CARTESIAN_POINT ( 'NONE',  ( -2.775557561562891351E-14, 19.94802294027085310, 18.49999999999999645 ) ) ;
#10513=AXIS2_PLACEMENT_3D ( 'NONE', #36288, #33281, #28717 ) ;
#10528=DIRECTION ( 'NONE',  ( 0.000000000000000000, 0.4999999999999953926, 0.8660254037844412611 ) ) ;
#10545=VECTOR ( 'NONE', #6618, 1000.000000000000000 ) ;
#10557=ORIENTED_EDGE ( 'NONE', *, *, #35957, .T. ) ;
#10568=ORIENTED_EDGE ( 'NONE', *, *, #28729, .F. ) ;
#10573=AXIS2_PLACEMENT_3D ( 'NONE', #19395, #16948, #22387 ) ;
#10628=ORIENTED_EDGE ( 'NONE', *, *, #12627, .T. ) ;
#10673=CARTESIAN_POINT ( 'NONE',  ( 3.368272016354702636, 101.4480229402710592, 32.49999999999999289 ) ) ;
#10687=( BOUNDED_CURVE ( )  B_SPLINE_CURVE ( 3, ( #20613, #3585, #576, #750 ),
 .UNSPECIFIED., .F., .T. ) 
 B_SPLINE_CURVE_WITH_KNOTS ( ( 4, 4 ),
 ( 4.712388980384679016, 6.283185307179586232 ),
 .UNSPECIFIED. ) 
 CURVE ( )  GEOMETRIC_REPRESENTATION_ITEM ( )  RATIONAL_B_SPLINE_CURVE ( ( 1.000000000000000000, 0.8047378541243626060, 0.8047378541243626060, 1.000000000000000000 ) ) 
 REPRESENTATION_ITEM ( '' )  );
#10693=DIRECTION ( 'NONE',  ( -1.000000000000000000, 0.000000000000000000, 0.000000000000000000 ) ) ;
#10722=EDGE_CURVE ( 'NONE', #34855, #20688, #3645, .T. ) ;
#10745=EDGE_LOOP ( 'NONE', ( #25544, #13582, #36950 ) ) ;
#10802=EDGE_CURVE ( 'NONE', #8343, #36432, #22456, .T. ) ;
#10852=VERTEX_POINT ( 'NONE', #1928 ) ;
#10891=ORIENTED_EDGE ( 'NONE', *, *, #34214, .T. ) ;
#10917=EDGE_CURVE ( 'NONE', #28376, #29465, #24881, .T. ) ;
#10936=ADVANCED_FACE ( 'NONE', ( #18639 ), #9807, .T. ) ;
#10977=EDGE_CURVE ( 'NONE', #21860, #27057, #27987, .T. ) ;
#10985=CARTESIAN_POINT ( 'NONE',  ( -37.50000000000000000, 103.4105893997321886, 27.49999999999999645 ) ) ;
#11048=LINE ( 'NONE', #5066, #13596 ) ;
#11094=CARTESIAN_POINT ( 'NONE',  ( 0.000000000000000000, 89.94802294027088863, 30.49999999999999289 ) ) ;
#11095=COLOUR_RGB ( '', 0.31764706, 0.68627451, 0.89019608) ;
#11098=ORIENTED_EDGE ( 'NONE', *, *, #8945, .T. ) ;
#11102=AXIS2_PLACEMENT_3D ( 'NONE', #14524, #17164, #3267 ) ;
#11133=AXIS2_PLACEMENT_3D ( 'NONE', #2180, #33315, #30509 ) ;
#11146=AXIS2_PLACEMENT_3D ( 'NONE', #33204, #1518, #27595 ) ;
#11179=AXIS2_PLACEMENT_3D ( 'NONE', #14850, #20637, #34912 ) ;
#11196=AXIS2_PLACEMENT_3D ( 'NONE', #22822, #31241, #36871 ) ;
#11201=DIRECTION ( 'NONE',  ( 1.224646799147353207E-16, 1.000000000000000000, -0.000000000000000000 ) ) ;
#11231=ORIENTED_EDGE ( 'NONE', *, *, #33143, .F. ) ;
#11232=CARTESIAN_POINT ( 'NONE',  ( -2.775557561562891351E-14, 19.94802294027085310, 27.49999999999999645 ) ) ;
#11240=EDGE_CURVE ( 'NONE', #6874, #374, #5300, .T. ) ;
#11273=DIRECTION ( 'NONE',  ( 0.000000000000000000, 0.4999999999999953926, -0.8660254037844412611 ) ) ;
#11288=AXIS2_PLACEMENT_3D ( 'NONE', #7432, #1619, #15873 ) ;
#11296=AXIS2_PLACEMENT_3D ( 'NONE', #17455, #11622, #23076 ) ;
#11314=CARTESIAN_POINT ( 'NONE',  ( 0.000000000000000000, 89.94802294027088863, -19.99999999999999645 ) ) ;
#11322=CARTESIAN_POINT ( 'NONE',  ( 17.55872235085559652, 89.94802294027088863, -24.99999999999999645 ) ) ;
#11324=DIRECTION ( 'NONE',  ( 0.000000000000000000, 0.000000000000000000, -1.000000000000000000 ) ) ;
#11463=EDGE_CURVE ( 'NONE', #4556, #8464, #33952, .T. ) ;
#11470=CARTESIAN_POINT ( 'NONE',  ( -28.99999999999999289, 103.4105893997321886, -19.99999999999999645 ) ) ;
#11485=DIRECTION ( 'NONE',  ( 0.000000000000000000, 0.000000000000000000, -1.000000000000000000 ) ) ;
#11493=EDGE_CURVE ( 'NONE', #6819, #15973, #13701, .T. ) ;
#11555=DIRECTION ( 'NONE',  ( -1.000000000000000000, 0.000000000000000000, 0.000000000000000000 ) ) ;
#11562=ORIENTED_EDGE ( 'NONE', *, *, #33038, .F. ) ;
#11589=( NAMED_UNIT ( * ) SI_UNIT ( $, .STERADIAN. ) SOLID_ANGLE_UNIT ( ) );
#11591=LINE ( 'NONE', #35251, #4479 ) ;
#11609=DIRECTION ( 'NONE',  ( -0.000000000000000000, -0.000000000000000000, -1.000000000000000000 ) ) ;
#11616=AXIS2_PLACEMENT_3D ( 'NONE', #22080, #31239, #2187 ) ;
#11622=DIRECTION ( 'NONE',  ( 0.000000000000000000, 0.000000000000000000, -1.000000000000000000 ) ) ;
#11629=CARTESIAN_POINT ( 'NONE',  ( 0.000000000000000000, 89.94802294027088863, -23.27834620192013304 ) ) ;
#11634=ORIENTED_EDGE ( 'NONE', *, *, #29123, .F. ) ;
#11658=EDGE_CURVE ( 'NONE', #22247, #24345, #35863, .T. ) ;
#11659=CARTESIAN_POINT ( 'NONE',  ( 0.000000000000000000, 89.94802294027088863, 27.49999999999999645 ) ) ;
#11687=CIRCLE ( 'NONE', #17690, 30.00000000000001421 ) ;
#11694=FACE_OUTER_BOUND ( 'NONE', #28773, .T. ) ;
#11711=LINE ( 'NONE', #1027, #19136 ) ;
#11716=ORIENTED_EDGE ( 'NONE', *, *, #33042, .T. ) ;
#11734=ADVANCED_FACE ( 'NONE', ( #12706 ), #29975, .T. ) ;
#11763=CARTESIAN_POINT ( 'NONE',  ( -37.50000000000000000, 103.4105893997321886, -19.99999999999999645 ) ) ;
#11784=DIRECTION ( 'NONE',  ( 1.000000000000000000, 0.000000000000000000, 0.000000000000000000 ) ) ;
#11800=DIRECTION ( 'NONE',  ( 0.000000000000000000, 0.4999999999999953926, 0.8660254037844412611 ) ) ;
#11808=EDGE_LOOP ( 'NONE', ( #30782, #6258, #24348, #15052, #1531, #15638, #4167, #24906, #35974, #10557, #30982, #20568 ) ) ;
#11816=APPLICATION_CONTEXT ( 'automotive_design' ) ;
#11834=ORIENTED_EDGE ( 'NONE', *, *, #24207, .T. ) ;
#11940=AXIS2_PLACEMENT_3D ( 'NONE', #14004, #5768, #14562 ) ;
#11963=DIRECTION ( 'NONE',  ( -1.000000000000000000, 0.000000000000000000, 0.000000000000000000 ) ) ;
#12023=CARTESIAN_POINT ( 'NONE',  ( 42.97377950131529190, 96.90768712682505281, 18.49999999999999645 ) ) ;
#12086=EDGE_CURVE ( 'NONE', #9029, #33241, #28636, .T. ) ;
#12182=ORIENTED_EDGE ( 'NONE', *, *, #31104, .F. ) ;
#12258=EDGE_CURVE ( 'NONE', #17955, #10852, #18306, .T. ) ;
#12352=CARTESIAN_POINT ( 'NONE',  ( 5.750000000000035527, 83.21147890756138565, -24.99999999999999289 ) ) ;
#12378=VERTEX_POINT ( 'NONE', #30665 ) ;
#12492=ORIENTED_EDGE ( 'NONE', *, *, #20477, .T. ) ;
#12493=DIRECTION ( 'NONE',  ( 0.000000000000000000, 0.4999999999999951150, -0.8660254037844414832 ) ) ;
#12496=DIRECTION ( 'NONE',  ( -1.000000000000000000, 0.000000000000000000, 0.000000000000000000 ) ) ;
#12501=ORIENTED_EDGE ( 'NONE', *, *, #25265, .T. ) ;
#12508=DIRECTION ( 'NONE',  ( 0.000000000000000000, -0.8660254037844421493, -0.4999999999999942268 ) ) ;
#12521=DIRECTION ( 'NONE',  ( 0.000000000000000000, 0.4999999999999951150, -0.8660254037844414832 ) ) ;
#12582=EDGE_CURVE ( 'NONE', #6533, #6253, #15083, .T. ) ;
#12594=DIRECTION ( 'NONE',  ( -1.000000000000000000, 0.000000000000000000, 0.000000000000000000 ) ) ;
#12615=VERTEX_POINT ( 'NONE', #29685 ) ;
#12627=EDGE_CURVE ( 'NONE', #755, #623, #29341, .T. ) ;
#12675=DIRECTION ( 'NONE',  ( -0.000000000000000000, -0.000000000000000000, -1.000000000000000000 ) ) ;
#12689=SURFACE_STYLE_FILL_AREA ( #15530 ) ;
#12700=VERTEX_POINT ( 'NONE', #34677 ) ;
#12704=AXIS2_PLACEMENT_3D ( 'NONE', #175, #34506, #8814 ) ;
#12706=FACE_OUTER_BOUND ( 'NONE', #8360, .T. ) ;
#12707=ADVANCED_FACE ( 'NONE', ( #705 ), #17767, .F. ) ;
#12755=AXIS2_PLACEMENT_3D ( 'NONE', #18616, #6422, #12594 ) ;
#12758=CYLINDRICAL_SURFACE ( 'NONE', #17484, 8.500000000000000000 ) ;
#12765=ADVANCED_FACE ( 'NONE', ( #23777 ), #29557, .F. ) ;
#12769=PLANE ( 'NONE',  #19576 ) ;
#12789=CARTESIAN_POINT ( 'NONE',  ( -3.368272016354731502, 78.44802294027070388, 32.49999999999999289 ) ) ;
#12843=CARTESIAN_POINT ( 'NONE',  ( -20.00000000000001066, 89.94802294027088863, 27.49999999999999645 ) ) ;
#12845=( BOUNDED_CURVE ( )  B_SPLINE_CURVE ( 3, ( #6384, #6753, #18186, #29615 ),
 .UNSPECIFIED., .F., .F. ) 
 B_SPLINE_CURVE_WITH_KNOTS ( ( 4, 4 ),
 ( 1.570796326794896558, 3.141592653589793116 ),
 .UNSPECIFIED. ) 
 CURVE ( )  GEOMETRIC_REPRESENTATION_ITEM ( )  RATIONAL_B_SPLINE_CURVE ( ( 1.000000000000000000, 0.8047378541243649375, 0.8047378541243649375, 1.000000000000000000 ) ) 
 REPRESENTATION_ITEM ( '' )  );
#12897=DIRECTION ( 'NONE',  ( 0.000000000000000000, -0.000000000000000000, 1.000000000000000000 ) ) ;
#12936=( GEOMETRIC_REPRESENTATION_CONTEXT ( 3 ) GLOBAL_UNCERTAINTY_ASSIGNED_CONTEXT ( ( #28668 ) ) GLOBAL_UNIT_ASSIGNED_CONTEXT ( ( #25495, #5613, #11589 ) ) REPRESENTATION_CONTEXT ( 'NONE', 'WORKASPACE' ) );
#12942=VECTOR ( 'NONE', #36818, 1000.000000000000000 ) ;
#12948=EDGE_CURVE ( 'NONE', #3254, #6819, #13087, .T. ) ;
#12963=LINE ( 'NONE', #27412, #10418 ) ;
#13011=DIRECTION ( 'NONE',  ( -0.7650473262243666639, 0.6439740589782693148, -0.000000000000000000 ) ) ;
#13087=( BOUNDED_CURVE ( )  B_SPLINE_CURVE ( 3, ( #17332, #74, #2193, #31742 ),
 .UNSPECIFIED., .F., .F. ) 
 B_SPLINE_CURVE_WITH_KNOTS ( ( 4, 4 ),
 ( 1.570796326794896558, 3.141592653589793116 ),
 .UNSPECIFIED. ) 
 CURVE ( )  GEOMETRIC_REPRESENTATION_ITEM ( )  RATIONAL_B_SPLINE_CURVE ( ( 1.000000000000000000, 0.8047378541243649375, 0.8047378541243649375, 1.000000000000000000 ) ) 
 REPRESENTATION_ITEM ( '' )  );
#13136=CIRCLE ( 'NONE', #4769, 8.500000000000007105 ) ;
#13140=ORIENTED_EDGE ( 'NONE', *, *, #30948, .T. ) ;
#13169=ORIENTED_EDGE ( 'NONE', *, *, #12086, .F. ) ;
#13200=ORIENTED_EDGE ( 'NONE', *, *, #2945, .T. ) ;
#13232=CARTESIAN_POINT ( 'NONE',  ( -46.00000000000000000, 103.4105893997321886, -19.99999999999999645 ) ) ;
#13277=CARTESIAN_POINT ( 'NONE',  ( -19.53925848833874213, 89.94802294027088863, 30.77834620192012594 ) ) ;
#13297=ADVANCED_FACE ( 'NONE', ( #17623 ), #36979, .T. ) ;
#13328=CARTESIAN_POINT ( 'NONE',  ( -19.31922176934808633, 76.99660315353983719, 27.49999999999999645 ) ) ;
#13491=ORIENTED_EDGE ( 'NONE', *, *, #2294, .F. ) ;
#13494=EDGE_CURVE ( 'NONE', #26470, #14180, #12845, .T. ) ;
#13495=CARTESIAN_POINT ( 'NONE',  ( 20.00000000000001066, 89.94802294027088863, -19.99999999999999645 ) ) ;
#13519=ORIENTED_EDGE ( 'NONE', *, *, #8071, .F. ) ;
#13530=EDGE_LOOP ( 'NONE', ( #5849, #18187 ) ) ;
#13572=EDGE_CURVE ( 'NONE', #27735, #33050, #26903, .T. ) ;
#13582=ORIENTED_EDGE ( 'NONE', *, *, #11493, .T. ) ;
#13596=VECTOR ( 'NONE', #36583, 1000.000000000000000 ) ;
#13598=CARTESIAN_POINT ( 'NONE',  ( 0.000000000000000000, 98.60827697811544112, 27.49999999999999645 ) ) ;
#13622=MECHANICAL_DESIGN_GEOMETRIC_PRESENTATION_REPRESENTATION('',(#5256),#12936);
#13652=AXIS2_PLACEMENT_3D ( 'NONE', #28173, #2492, #13914 ) ;
#13656=VERTEX_POINT ( 'NONE', #7319 ) ;
#13701=LINE ( 'NONE', #14050, #15488 ) ;
#13710=CARTESIAN_POINT ( 'NONE',  ( 0.000000000000000000, 101.4480229402710734, 32.49999999999999289 ) ) ;
#13749=DIRECTION ( 'NONE',  ( 0.000000000000000000, 0.4999999999999944489, 0.8660254037844418162 ) ) ;
#13818=ORIENTED_EDGE ( 'NONE', *, *, #21012, .T. ) ;
#13839=ORIENTED_EDGE ( 'NONE', *, *, #17869, .F. ) ;
#13875=ORIENTED_EDGE ( 'NONE', *, *, #25205, .F. ) ;
#13876=ORIENTED_EDGE ( 'NONE', *, *, #12258, .F. ) ;
#13914=DIRECTION ( 'NONE',  ( 0.000000000000000000, 0.4999999999999953926, 0.8660254037844412611 ) ) ;
#13926=EDGE_CURVE ( 'NONE', #21384, #15883, #33498, .T. ) ;
#13946=VERTEX_POINT ( 'NONE', #20769 ) ;
#13969=DIRECTION ( 'NONE',  ( -0.000000000000000000, -0.000000000000000000, 1.000000000000000000 ) ) ;
#14004=CARTESIAN_POINT ( 'NONE',  ( -37.50000000000000000, 103.4105893997321886, -19.99999999999999645 ) ) ;
#14027=DIRECTION ( 'NONE',  ( 0.000000000000000000, 0.4999999999999953926, 0.8660254037844412611 ) ) ;
#14043=( NAMED_UNIT ( * ) SI_UNIT ( $, .STERADIAN. ) SOLID_ANGLE_UNIT ( ) );
#14050=CARTESIAN_POINT ( 'NONE',  ( 0.000000000000000000, 101.4832769781154127, 32.47964607176053420 ) ) ;
#14072=AXIS2_PLACEMENT_3D ( 'NONE', #4257, #15865, #33104 ) ;
#14085=CIRCLE ( 'NONE', #24294, 3.500000000000003109 ) ;
#14093=DIRECTION ( 'NONE',  ( -0.000000000000000000, -0.8660254037844420383, -0.4999999999999941713 ) ) ;
#14112=DIRECTION ( 'NONE',  ( -1.000000000000000000, 0.000000000000000000, 0.000000000000000000 ) ) ;
#14180=VERTEX_POINT ( 'NONE', #5206 ) ;
#14183=( NAMED_UNIT ( * ) SI_UNIT ( $, .STERADIAN. ) SOLID_ANGLE_UNIT ( ) );
#14248=( NAMED_UNIT ( * ) PLANE_ANGLE_UNIT ( ) SI_UNIT ( $, .RADIAN. ) );
#14323=CARTESIAN_POINT ( 'NONE',  ( 19.31922176934805435, 76.99660315353983719, 27.49999999999999645 ) ) ;
#14518=DIRECTION ( 'NONE',  ( 0.000000000000000000, 0.4999999999999959477, -0.8660254037844409281 ) ) ;
#14524=CARTESIAN_POINT ( 'NONE',  ( 37.50000000000000000, 103.4105893997321743, -19.99999999999999645 ) ) ;
#14539=ORIENTED_EDGE ( 'NONE', *, *, #10722, .T. ) ;
#14549=ORIENTED_EDGE ( 'NONE', *, *, #10351, .F. ) ;
#14562=DIRECTION ( 'NONE',  ( 1.000000000000000000, 0.000000000000000000, 0.000000000000000000 ) ) ;
#14622=ORIENTED_EDGE ( 'NONE', *, *, #6710, .F. ) ;
#14666=CARTESIAN_POINT ( 'NONE',  ( 42.97377950131529190, 96.90768712682505281, 27.49999999999999645 ) ) ;
#14700=CYLINDRICAL_SURFACE ( 'NONE', #11102, 3.500000000000003109 ) ;
#14734=ORIENTED_EDGE ( 'NONE', *, *, #10802, .T. ) ;
#14773=DIRECTION ( 'NONE',  ( -0.7650473262243665529, 0.6439740589782693148, 0.000000000000000000 ) ) ;
#14783=EDGE_CURVE ( 'NONE', #30183, #4131, #20365, .T. ) ;
#14804=EDGE_LOOP ( 'NONE', ( #13200, #4812 ) ) ;
#14826=LINE ( 'NONE', #20818, #3871 ) ;
#14837=EDGE_CURVE ( 'NONE', #6533, #7296, #32876, .T. ) ;
#14847=DIRECTION ( 'NONE',  ( 0.000000000000000000, 0.000000000000000000, -1.000000000000000000 ) ) ;
#14850=CARTESIAN_POINT ( 'NONE',  ( 0.000000000000000000, 85.61789592134881843, -27.49999999999990408 ) ) ;
#14869=AXIS2_PLACEMENT_3D ( 'NONE', #21169, #6923, #3739 ) ;
#14876=AXIS2_PLACEMENT_3D ( 'NONE', #1911, #35866, #10528 ) ;
#15052=ORIENTED_EDGE ( 'NONE', *, *, #23717, .F. ) ;
#15074=CARTESIAN_POINT ( 'NONE',  ( 20.00000000000001066, 89.94802294027088863, -19.99999999999999645 ) ) ;
#15083=LINE ( 'NONE', #9650, #21565 ) ;
#15128=EDGE_CURVE ( 'NONE', #36148, #4050, #19734, .T. ) ;
#15161=ORIENTED_EDGE ( 'NONE', *, *, #31933, .F. ) ;
#15196=LINE ( 'NONE', #4151, #3362 ) ;
#15214=FACE_OUTER_BOUND ( 'NONE', #32479, .T. ) ;
#15215=DIRECTION ( 'NONE',  ( 0.000000000000000000, -0.8660254037844418162, 0.4999999999999945044 ) ) ;
#15238=VERTEX_POINT ( 'NONE', #856 ) ;
#15255=AXIS2_PLACEMENT_3D ( 'NONE', #34491, #28841, #8800 ) ;
#15356=ORIENTED_EDGE ( 'NONE', *, *, #19200, .F. ) ;
#15359=EDGE_LOOP ( 'NONE', ( #3909, #21880, #1190, #28404, #21052, #34875, #27840, #30152 ) ) ;
#15373=ORIENTED_EDGE ( 'NONE', *, *, #17442, .T. ) ;
#15488=VECTOR ( 'NONE', #8444, 1000.000000000000114 ) ;
#15491=EDGE_CURVE ( 'NONE', #36272, #24938, #18563, .T. ) ;
#15493=ORIENTED_EDGE ( 'NONE', *, *, #35963, .T. ) ;
#15503=DIRECTION ( 'NONE',  ( -0.000000000000000000, -0.000000000000000000, 1.000000000000000000 ) ) ;
#15504=VECTOR ( 'NONE', #29633, 999.9999999999998863 ) ;
#15506=DIRECTION ( 'NONE',  ( -0.7650473262243671080, -0.6439740589782688707, -0.000000000000000000 ) ) ;
#15530=FILL_AREA_STYLE ('',( #4094 ) ) ;
#15562=CIRCLE ( 'NONE', #20940, 19.53925848833874213 ) ;
#15604=DIRECTION ( 'NONE',  ( 1.000000000000000000, 0.000000000000000000, 0.000000000000000000 ) ) ;
#15637=ORIENTED_EDGE ( 'NONE', *, *, #23774, .F. ) ;
#15638=ORIENTED_EDGE ( 'NONE', *, *, #13926, .F. ) ;
#15696=CARTESIAN_POINT ( 'NONE',  ( -2.448772250512182280E-15, 99.94802294027086020, -19.99999999999999645 ) ) ;
#15699=ORIENTED_EDGE ( 'NONE', *, *, #16710, .T. ) ;
#15702=DIRECTION ( 'NONE',  ( -0.000000000000000000, -0.000000000000000000, 1.000000000000000000 ) ) ;
#15717=ORIENTED_EDGE ( 'NONE', *, *, #18375, .F. ) ;
#15747=ORIENTED_EDGE ( 'NONE', *, *, #31672, .T. ) ;
#15748=EDGE_CURVE ( 'NONE', #4556, #3254, #34881, .T. ) ;
#15865=DIRECTION ( 'NONE',  ( -0.000000000000000000, -0.8660254037844419273, -0.4999999999999941158 ) ) ;
#15873=DIRECTION ( 'NONE',  ( 1.000000000000000000, 0.000000000000000000, 0.000000000000000000 ) ) ;
#15883=VERTEX_POINT ( 'NONE', #28340 ) ;
#15916=ORIENTED_EDGE ( 'NONE', *, *, #25265, .F. ) ;
#15929=EDGE_CURVE ( 'NONE', #28764, #8464, #33412, .T. ) ;
#15971=FACE_OUTER_BOUND ( 'NONE', #29519, .T. ) ;
#15973=VERTEX_POINT ( 'NONE', #22127 ) ;
#15978=PRODUCT_DEFINITION ( 'UNKNOWN', '', #23146, #16694 ) ;
#16022=DIRECTION ( 'NONE',  ( 0.000000000000000000, -0.8660254037844419273, -0.4999999999999945044 ) ) ;
#16036=ORIENTED_EDGE ( 'NONE', *, *, #20828, .T. ) ;
#16040=VECTOR ( 'NONE', #19773, 1000.000000000000000 ) ;
#16059=CARTESIAN_POINT ( 'NONE',  ( 28.99999999999998934, 103.4105893997321743, -11.00000000000000355 ) ) ;
#16064=ADVANCED_FACE ( 'NONE', ( #16139 ), #1871, .T. ) ;
#16066=CARTESIAN_POINT ( 'NONE',  ( 19.31922176934805435, 76.99660315353983719, 27.49999999999999645 ) ) ;
#16073=DIRECTION ( 'NONE',  ( 0.000000000000000000, -0.8660254037844421493, -0.4999999999999942268 ) ) ;
#16092=CARTESIAN_POINT ( 'NONE',  ( 3.368272016354702636, 101.4480229402710592, -25.00000000000000000 ) ) ;
#16105=TOROIDAL_SURFACE ( 'NONE', #25078, 17.55872235085559652, 2.000000000000000000 ) ;
#16123=EDGE_LOOP ( 'NONE', ( #15717, #34697, #32342, #8153, #27013, #16395, #22197, #19704 ) ) ;
#16129=AXIS2_PLACEMENT_3D ( 'NONE', #36384, #25142, #10693 ) ;
#16139=FACE_OUTER_BOUND ( 'NONE', #15359, .T. ) ;
#16172=FACE_OUTER_BOUND ( 'NONE', #23912, .T. ) ;
#16186=ORIENTED_EDGE ( 'NONE', *, *, #12582, .F. ) ;
#16371=DIRECTION ( 'NONE',  ( -1.000000000000000000, 0.000000000000000000, 0.000000000000000000 ) ) ;
#16395=ORIENTED_EDGE ( 'NONE', *, *, #10977, .F. ) ;
#16397=VECTOR ( 'NONE', #28505, 1000.000000000000000 ) ;
#16422=ORIENTED_EDGE ( 'NONE', *, *, #20999, .T. ) ;
#16432=ORIENTED_EDGE ( 'NONE', *, *, #12948, .T. ) ;
#16518=CARTESIAN_POINT ( 'NONE',  ( 0.000000000000000000, 89.94802294027088863, 30.77834620192012594 ) ) ;
#16521=FACE_OUTER_BOUND ( 'NONE', #25321, .T. ) ;
#16532=VERTEX_POINT ( 'NONE', #17112 ) ;
#16534=ADVANCED_FACE ( 'NONE', ( #19755 ), #16105, .T. ) ;
#16603=DIRECTION ( 'NONE',  ( -0.000000000000000000, -0.8660254037844414832, 0.4999999999999953371 ) ) ;
#16668=AXIS2_PLACEMENT_3D ( 'NONE', #21243, #32884, #29878 ) ;
#16694=PRODUCT_DEFINITION_CONTEXT ( 'detailed design', #11816, 'design' ) ;
#16710=EDGE_CURVE ( 'NONE', #18201, #12378, #6216, .T. ) ;
#16729=FACE_OUTER_BOUND ( 'NONE', #26619, .T. ) ;
#16774=DIRECTION ( 'NONE',  ( 1.000000000000000000, 0.000000000000000000, 0.000000000000000000 ) ) ;
#16826=DIRECTION ( 'NONE',  ( -1.000000000000000000, 0.000000000000000000, 0.000000000000000000 ) ) ;
#16948=DIRECTION ( 'NONE',  ( 0.000000000000000000, -0.8660254037844420383, -0.4999999999999945599 ) ) ;
#16958=VERTEX_POINT ( 'NONE', #9124 ) ;
#17022=DIRECTION ( 'NONE',  ( -1.000000000000000000, 0.000000000000000000, 0.000000000000000000 ) ) ;
#17035=DIRECTION ( 'NONE',  ( 0.000000000000000000, -0.8660254037844419273, 0.4999999999999945599 ) ) ;
#17065=DIRECTION ( 'NONE',  ( 0.000000000000000000, 0.4999999999999951150, -0.8660254037844414832 ) ) ;
#17089=DIRECTION ( 'NONE',  ( 1.000000000000000000, 0.000000000000000000, 0.000000000000000000 ) ) ;
#17090=DIRECTION ( 'NONE',  ( 1.000000000000000000, 0.000000000000000000, -0.000000000000000000 ) ) ;
#17112=CARTESIAN_POINT ( 'NONE',  ( 20.00000000000001066, 89.94802294027088863, 27.49999999999999645 ) ) ;
#17152=DIRECTION ( 'NONE',  ( 0.000000000000000000, 0.4999999999999953926, 0.8660254037844412611 ) ) ;
#17153=CARTESIAN_POINT ( 'NONE',  ( 0.000000000000000000, 85.61789592134881843, -27.49999999999990408 ) ) ;
#17164=DIRECTION ( 'NONE',  ( -0.000000000000000000, -0.000000000000000000, 1.000000000000000000 ) ) ;
#17173=CARTESIAN_POINT ( 'NONE',  ( 0.000000000000000000, 89.94802294027088863, -19.99999999999999645 ) ) ;
#17199=EDGE_CURVE ( 'NONE', #530, #28731, #20757, .T. ) ;
#17210=DIRECTION ( 'NONE',  ( -0.000000000000000000, 0.8660254037844420383, -0.4999999999999945599 ) ) ;
#17244=ORIENTED_EDGE ( 'NONE', *, *, #15929, .F. ) ;
#17245=AXIS2_PLACEMENT_3D ( 'NONE', #10485, #19310, #33374 ) ;
#17248=ORIENTED_EDGE ( 'NONE', *, *, #17869, .T. ) ;
#17253=LINE ( 'NONE', #19326, #31958 ) ;
#17322=LINE ( 'NONE', #5512, #16040 ) ;
#17327=AXIS2_PLACEMENT_3D ( 'NONE', #3161, #34484, #20409 ) ;
#17332=CARTESIAN_POINT ( 'NONE',  ( -5.750000000000000000, 89.94802294027094547, 32.49999999999999289 ) ) ;
#17338=ORIENTED_EDGE ( 'NONE', *, *, #2252, .F. ) ;
#17387=DIRECTION ( 'NONE',  ( 1.000000000000000000, 0.000000000000000000, 0.000000000000000000 ) ) ;
#17398=DIRECTION ( 'NONE',  ( -0.000000000000000000, -0.8660254037844414832, -0.4999999999999953371 ) ) ;
#17442=EDGE_CURVE ( 'NONE', #24345, #12378, #17763, .T. ) ;
#17452=CARTESIAN_POINT ( 'NONE',  ( 0.000000000000000000, 81.28776890242660613, -29.99999999999987566 ) ) ;
#17455=CARTESIAN_POINT ( 'NONE',  ( -2.775557561562891351E-14, 19.94802294027085310, 27.49999999999999645 ) ) ;
#17484=AXIS2_PLACEMENT_3D ( 'NONE', #3425, #3776, #15604 ) ;
#17555=CIRCLE ( 'NONE', #12755, 20.00000000000001066 ) ;
#17579=ORIENTED_EDGE ( 'NONE', *, *, #26581, .T. ) ;
#17597=ORIENTED_EDGE ( 'NONE', *, *, #12086, .T. ) ;
#17616=CARTESIAN_POINT ( 'NONE',  ( -40.98360655737705827, 111.1639425680974398, -19.99999999999999645 ) ) ;
#17623=FACE_OUTER_BOUND ( 'NONE', #30735, .T. ) ;
#17640=CARTESIAN_POINT ( 'NONE',  ( 17.55872235085560007, 89.94802294027088863, 30.49999999999999289 ) ) ;
#17648=CARTESIAN_POINT ( 'NONE',  ( -20.00000000000001066, 89.94802294027088863, -19.99999999999999645 ) ) ;
#17664=ORIENTED_EDGE ( 'NONE', *, *, #6151, .F. ) ;
#17667=CARTESIAN_POINT ( 'NONE',  ( -42.97377950131527058, 96.90768712682508124, 27.49999999999999645 ) ) ;
#17690=AXIS2_PLACEMENT_3D ( 'NONE', #8645, #22739, #17089 ) ;
#17710=DIRECTION ( 'NONE',  ( -1.000000000000000000, 0.000000000000000000, 0.000000000000000000 ) ) ;
#17763=CIRCLE ( 'NONE', #27354, 20.00000000000001066 ) ;
#17767=CYLINDRICAL_SURFACE ( 'NONE', #6, 3.500000000000003109 ) ;
#17833=CIRCLE ( 'NONE', #3476, 3.500000000000003109 ) ;
#17834=CIRCLE ( 'NONE', #2268, 8.500000000000003553 ) ;
#17869=EDGE_CURVE ( 'NONE', #12378, #20688, #8529, .T. ) ;
#17876=ADVANCED_FACE ( 'NONE', ( #22559 ), #34559, .T. ) ;
#17924=CARTESIAN_POINT ( 'NONE',  ( -5.750000000000036415, 83.21147890756139986, -24.99999999999999645 ) ) ;
#17952=CIRCLE ( 'NONE', #32918, 2.000000000000001776 ) ;
#17955=VERTEX_POINT ( 'NONE', #12023 ) ;
#18002=ADVANCED_FACE ( 'NONE', ( #15214 ), #12758, .T. ) ;
#18035=DIRECTION ( 'NONE',  ( -0.7650473262243671080, -0.6439740589782688707, 0.000000000000000000 ) ) ;
#18067=DIRECTION ( 'NONE',  ( 0.1391731009600657432, -1.704378926181559679E-17, 0.9902680687415703620 ) ) ;
#18108=ADVANCED_FACE ( 'NONE', ( #16521 ), #10316, .T. ) ;
#18111=PRODUCT_CONTEXT ( 'NONE', #26899, 'mechanical' ) ;
#18113=CYLINDRICAL_SURFACE ( 'NONE', #14072, 1.750000000000015765 ) ;
#18124=ORIENTED_EDGE ( 'NONE', *, *, #11240, .F. ) ;
#18156=CARTESIAN_POINT ( 'NONE',  ( -2.775557561562891351E-14, 19.94802294027085310, -11.00000000000000000 ) ) ;
#18186=CARTESIAN_POINT ( 'NONE',  ( -3.368272016354703968, 101.4480229402710592, -25.00000000000000000 ) ) ;
#18187=ORIENTED_EDGE ( 'NONE', *, *, #24410, .T. ) ;
#18201=VERTEX_POINT ( 'NONE', #9964 ) ;
#18211=CIRCLE ( 'NONE', #6225, 3.500000000000003109 ) ;
#18264=CYLINDRICAL_SURFACE ( 'NONE', #33716, 8.500000000000000000 ) ;
#18306=LINE ( 'NONE', #29733, #9541 ) ;
#18326=CARTESIAN_POINT ( 'NONE',  ( -42.97377950131527058, 96.90768712682508124, -19.99999999999999645 ) ) ;
#18375=EDGE_CURVE ( 'NONE', #19982, #755, #31289, .T. ) ;
#18376=CARTESIAN_POINT ( 'NONE',  ( 4.897544501024384282E-15, 69.94802294027087441, 27.49999999999999645 ) ) ;
#18453=DIRECTION ( 'NONE',  ( 1.000000000000000000, 0.000000000000000000, 0.000000000000000000 ) ) ;
#18475=DIRECTION ( 'NONE',  ( -0.000000000000000000, -0.000000000000000000, 1.000000000000000000 ) ) ;
#18481=EDGE_LOOP ( 'NONE', ( #13876, #1509, #32130, #30081 ) ) ;
#18529=DIRECTION ( 'NONE',  ( 0.000000000000000000, 0.4999999999999959477, -0.8660254037844409281 ) ) ;
#18543=EDGE_LOOP ( 'NONE', ( #3404, #8595, #31456, #16186, #21857 ) ) ;
#18560=ORIENTED_EDGE ( 'NONE', *, *, #29374, .T. ) ;
#18563=CIRCLE ( 'NONE', #2398, 1.750000000000015765 ) ;
#18616=CARTESIAN_POINT ( 'NONE',  ( 0.000000000000000000, 89.94802294027088863, 27.49999999999999645 ) ) ;
#18639=FACE_OUTER_BOUND ( 'NONE', #1925, .T. ) ;
#18687=CARTESIAN_POINT ( 'NONE',  ( -46.00000000000000000, 103.4105893997321886, -19.99999999999999645 ) ) ;
#18763=ADVANCED_FACE ( 'NONE', ( #21466 ), #32903, .F. ) ;
#18799=ADVANCED_FACE ( 'NONE', ( #32141 ), #18264, .T. ) ;
#18819=DIRECTION ( 'NONE',  ( -1.000000000000000000, 0.000000000000000000, 0.000000000000000000 ) ) ;
#18822=EDGE_CURVE ( 'NONE', #36472, #12700, #9148, .T. ) ;
#18853=ORIENTED_EDGE ( 'NONE', *, *, #30286, .F. ) ;
#18873=AXIS2_PLACEMENT_3D ( 'NONE', #9088, #26706, #17710 ) ;
#18980=CONICAL_SURFACE ( 'NONE', #5217, 20.00000000000001066, 0.1396263401595466691 ) ;
#19018=EDGE_CURVE ( 'NONE', #19694, #29078, #24151, .T. ) ;
#19129=ORIENTED_EDGE ( 'NONE', *, *, #20881, .F. ) ;
#19136=VECTOR ( 'NONE', #32138, 1000.000000000000000 ) ;
#19152=ORIENTED_EDGE ( 'NONE', *, *, #6710, .T. ) ;
#19200=EDGE_CURVE ( 'NONE', #16532, #19694, #17555, .T. ) ;
#19300=CARTESIAN_POINT ( 'NONE',  ( 5.750000000000000000, 89.94802294027094547, 32.49999999999999289 ) ) ;
#19310=DIRECTION ( 'NONE',  ( 0.000000000000000000, 0.000000000000000000, -1.000000000000000000 ) ) ;
#19326=CARTESIAN_POINT ( 'NONE',  ( 2.143131898507887033E-16, 84.74289592134881843, -25.98445554337711627 ) ) ;
#19330=EDGE_CURVE ( 'NONE', #14180, #6533, #12963, .T. ) ;
#19395=CARTESIAN_POINT ( 'NONE',  ( 0.000000000000000000, 89.94802294027094547, -24.99999999999999645 ) ) ;
#19407=EDGE_CURVE ( 'NONE', #15883, #21230, #25884, .T. ) ;
#19435=EDGE_LOOP ( 'NONE', ( #33789, #5900, #3550, #6982 ) ) ;
#19489=DIRECTION ( 'NONE',  ( 1.000000000000000000, 0.000000000000000000, 0.000000000000000000 ) ) ;
#19514=STYLED_ITEM ( 'NONE', ( #26960 ), #32508 ) ;
#19529=ORIENTED_EDGE ( 'NONE', *, *, #21027, .T. ) ;
#19535=ORIENTED_EDGE ( 'NONE', *, *, #4827, .F. ) ;
#19536=DIRECTION ( 'NONE',  ( -1.000000000000000000, 0.000000000000000000, 0.000000000000000000 ) ) ;
#19576=AXIS2_PLACEMENT_3D ( 'NONE', #30210, #33037, #35321 ) ;
#19591=CARTESIAN_POINT ( 'NONE',  ( -42.97377950131527058, 96.90768712682508124, -19.99999999999999645 ) ) ;
#19603=DIRECTION ( 'NONE',  ( 0.000000000000000000, -0.8660254037844421493, -0.4999999999999942268 ) ) ;
#19633=LINE ( 'NONE', #28243, #30391 ) ;
#19644=VECTOR ( 'NONE', #18035, 1000.000000000000000 ) ;
#19687=EDGE_CURVE ( 'NONE', #7296, #3432, #20510, .T. ) ;
#19694=VERTEX_POINT ( 'NONE', #18376 ) ;
#19704=ORIENTED_EDGE ( 'NONE', *, *, #33576, .F. ) ;
#19734=CIRCLE ( 'NONE', #5977, 100.0000000000000142 ) ;
#19755=FACE_OUTER_BOUND ( 'NONE', #9034, .T. ) ;
#19759=CARTESIAN_POINT ( 'NONE',  ( -37.50000000000000000, 103.4105893997321886, 27.49999999999999645 ) ) ;
#19772=ORIENTED_EDGE ( 'NONE', *, *, #18822, .F. ) ;
#19773=DIRECTION ( 'NONE',  ( -0.7650473262243671080, -0.6439740589782688707, 0.000000000000000000 ) ) ;
#19829=EDGE_CURVE ( 'NONE', #35994, #28731, #24577, .T. ) ;
#19880=CARTESIAN_POINT ( 'NONE',  ( -5.750000000000000000, 89.94802294027094547, -24.99999999999999645 ) ) ;
#19975=DIRECTION ( 'NONE',  ( 0.000000000000000000, 0.4999999999999951150, -0.8660254037844414832 ) ) ;
#19982=VERTEX_POINT ( 'NONE', #18687 ) ;
#20008=DIRECTION ( 'NONE',  ( 0.000000000000000000, 0.4999999999999953926, -0.8660254037844412611 ) ) ;
#20027=VERTEX_POINT ( 'NONE', #16066 ) ;
#20063=CARTESIAN_POINT ( 'NONE',  ( 0.000000000000000000, 89.94802294027097389, 32.49999999999990052 ) ) ;
#20070=DIRECTION ( 'NONE',  ( -0.000000000000000000, -0.000000000000000000, 1.000000000000000000 ) ) ;
#20083=DIRECTION ( 'NONE',  ( -0.000000000000000000, -0.000000000000000000, -1.000000000000000000 ) ) ;
#20103=CARTESIAN_POINT ( 'NONE',  ( 0.000000000000000000, 89.94802294027088863, -23.00000000000000000 ) ) ;
#20146=ORIENTED_EDGE ( 'NONE', *, *, #19018, .T. ) ;
#20181=VECTOR ( 'NONE', #1243, 1000.000000000000000 ) ;
#20230=PLANE ( 'NONE',  #20640 ) ;
#20243=LINE ( 'NONE', #721, #29586 ) ;
#20246=VERTEX_POINT ( 'NONE', #25799 ) ;
#20279=CARTESIAN_POINT ( 'NONE',  ( -40.98360655737706537, 111.1639425680974682, -11.00000000000000355 ) ) ;
#20294=FACE_OUTER_BOUND ( 'NONE', #25309, .T. ) ;
#20365=CIRCLE ( 'NONE', #17327, 17.55872235085559652 ) ;
#20391=CIRCLE ( 'NONE', #31161, 100.0000000000000142 ) ;
#20409=DIRECTION ( 'NONE',  ( -1.000000000000000000, 0.000000000000000000, 0.000000000000000000 ) ) ;
#20436=EDGE_LOOP ( 'NONE', ( #4651, #32690 ) ) ;
#20447=CARTESIAN_POINT ( 'NONE',  ( -42.97377950131527058, 96.90768712682508124, -11.00000000000000000 ) ) ;
#20477=EDGE_CURVE ( 'NONE', #24938, #25464, #43, .T. ) ;
#20480=ORIENTED_EDGE ( 'NONE', *, *, #8945, .F. ) ;
#20494=DIRECTION ( 'NONE',  ( 0.000000000000000000, 0.000000000000000000, -1.000000000000000000 ) ) ;
#20510=( BOUNDED_CURVE ( )  B_SPLINE_CURVE ( 3, ( #6933, #12352, #23823, #35275 ),
 .UNSPECIFIED., .F., .T. ) 
 B_SPLINE_CURVE_WITH_KNOTS ( ( 4, 4 ),
 ( 4.712388980384679016, 6.283185307179586232 ),
 .UNSPECIFIED. ) 
 CURVE ( )  GEOMETRIC_REPRESENTATION_ITEM ( )  RATIONAL_B_SPLINE_CURVE ( ( 1.000000000000000000, 0.8047378541243626060, 0.8047378541243626060, 1.000000000000000000 ) ) 
 REPRESENTATION_ITEM ( '' )  );
#20517=DIRECTION ( 'NONE',  ( 0.000000000000000000, 0.000000000000000000, -1.000000000000000000 ) ) ;
#20560=DIRECTION ( 'NONE',  ( 0.000000000000000000, 0.000000000000000000, -1.000000000000000000 ) ) ;
#20568=ORIENTED_EDGE ( 'NONE', *, *, #19200, .T. ) ;
#20613=CARTESIAN_POINT ( 'NONE',  ( 5.750000000000000000, 89.94802294027094547, 32.49999999999999289 ) ) ;
#20623=DIRECTION ( 'NONE',  ( -0.000000000000000000, -0.000000000000000000, 1.000000000000000000 ) ) ;
#20637=DIRECTION ( 'NONE',  ( -0.000000000000000000, -0.8660254037844419273, -0.4999999999999941158 ) ) ;
#20640=AXIS2_PLACEMENT_3D ( 'NONE', #11232, #22859, #19489 ) ;
#20647=LINE ( 'NONE', #29286, #5164 ) ;
#20651=VECTOR ( 'NONE', #18067, 999.9999999999998863 ) ;
#20673=MECHANICAL_DESIGN_GEOMETRIC_PRESENTATION_REPRESENTATION('',(#19514),#31457);
#20679=ORIENTED_EDGE ( 'NONE', *, *, #22949, .F. ) ;
#20688=VERTEX_POINT ( 'NONE', #13495 ) ;
#20757=CIRCLE ( 'NONE', #7576, 3.500000000000003109 ) ;
#20767=DIRECTION ( 'NONE',  ( 1.000000000000000000, 0.000000000000000000, 0.000000000000000000 ) ) ;
#20769=CARTESIAN_POINT ( 'NONE',  ( -42.97377950131527058, 96.90768712682508124, -19.99999999999999645 ) ) ;
#20818=CARTESIAN_POINT ( 'NONE',  ( 42.97377950131527058, 96.90768712682506703, 27.49999999999999645 ) ) ;
#20828=EDGE_CURVE ( 'NONE', #5579, #6874, #5649, .T. ) ;
#20859=CIRCLE ( 'NONE', #14869, 19.53925848833874213 ) ;
#20860=DIRECTION ( 'NONE',  ( 1.000000000000000000, 0.000000000000000000, 0.000000000000000000 ) ) ;
#20867=VECTOR ( 'NONE', #8238, 1000.000000000000000 ) ;
#20881=EDGE_CURVE ( 'NONE', #36272, #20246, #17253, .T. ) ;
#20888=AXIS2_PLACEMENT_3D ( 'NONE', #18156, #12897, #24554 ) ;
#20940=AXIS2_PLACEMENT_3D ( 'NONE', #16518, #21961, #21767 ) ;
#20999=EDGE_CURVE ( 'NONE', #13946, #4610, #11591, .T. ) ;
#21012=EDGE_CURVE ( 'NONE', #26378, #13656, #20243, .T. ) ;
#21027=EDGE_CURVE ( 'NONE', #35994, #6252, #31981, .T. ) ;
#21052=ORIENTED_EDGE ( 'NONE', *, *, #31417, .T. ) ;
#21073=DIRECTION ( 'NONE',  ( 0.000000000000000000, -0.8660254037844418162, -0.4999999999999945044 ) ) ;
#21122=CARTESIAN_POINT ( 'NONE',  ( 37.50000000000000000, 103.4105893997321743, 27.49999999999999645 ) ) ;
#21127=VECTOR ( 'NONE', #11324, 1000.000000000000000 ) ;
#21151=ORIENTED_EDGE ( 'NONE', *, *, #20999, .F. ) ;
#21156=CARTESIAN_POINT ( 'NONE',  ( 0.000000000000000000, 86.49289592134881843, -29.01554445662268833 ) ) ;
#21169=CARTESIAN_POINT ( 'NONE',  ( 0.000000000000000000, 89.94802294027088863, -23.27834620192013304 ) ) ;
#21200=ORIENTED_EDGE ( 'NONE', *, *, #15748, .T. ) ;
#21217=DIRECTION ( 'NONE',  ( 1.000000000000000000, 0.000000000000000000, 0.000000000000000000 ) ) ;
#21230=VERTEX_POINT ( 'NONE', #26974 ) ;
#21243=CARTESIAN_POINT ( 'NONE',  ( -2.775557561562891351E-14, 19.94802294027085310, -19.99999999999999645 ) ) ;
#21287=EDGE_CURVE ( 'NONE', #6253, #3167, #27238, .T. ) ;
#21354=CIRCLE ( 'NONE', #24962, 30.00000000000001421 ) ;
#21384=VERTEX_POINT ( 'NONE', #28632 ) ;
#21385=AXIS2_PLACEMENT_3D ( 'NONE', #8896, #30384, #36396 ) ;
#21400=ORIENTED_EDGE ( 'NONE', *, *, #24207, .F. ) ;
#21437=ORIENTED_EDGE ( 'NONE', *, *, #6151, .T. ) ;
#21444=CARTESIAN_POINT ( 'NONE',  ( 37.50000000000000000, 103.4105893997321743, -11.00000000000000355 ) ) ;
#21466=FACE_OUTER_BOUND ( 'NONE', #6938, .T. ) ;
#21519=DIRECTION ( 'NONE',  ( -0.000000000000000000, -0.000000000000000000, 1.000000000000000000 ) ) ;
#21560=CARTESIAN_POINT ( 'NONE',  ( 0.000000000000000000, 89.94802294027088863, -19.99999999999999645 ) ) ;
#21565=VECTOR ( 'NONE', #21073, 1000.000000000000114 ) ;
#21581=EDGE_CURVE ( 'NONE', #8343, #27735, #26746, .T. ) ;
#21583=ADVANCED_FACE ( 'NONE', ( #23950 ), #18113, .F. ) ;
#21641=DIRECTION ( 'NONE',  ( 0.000000000000000000, 0.4999999999999944489, -0.8660254037844418162 ) ) ;
#21694=DIRECTION ( 'NONE',  ( 1.000000000000000000, 0.000000000000000000, 0.000000000000000000 ) ) ;
#21724=ORIENTED_EDGE ( 'NONE', *, *, #15929, .T. ) ;
#21767=DIRECTION ( 'NONE',  ( -1.000000000000000000, 0.000000000000000000, 0.000000000000000000 ) ) ;
#21770=DIRECTION ( 'NONE',  ( 0.000000000000000000, -0.8660254037844418162, -0.4999999999999945044 ) ) ;
#21796=ORIENTED_EDGE ( 'NONE', *, *, #4596, .T. ) ;
#21799=DIRECTION ( 'NONE',  ( 0.000000000000000000, -0.000000000000000000, 1.000000000000000000 ) ) ;
#21802=ADVANCED_FACE ( 'NONE', ( #11694 ), #14700, .F. ) ;
#21805=CARTESIAN_POINT ( 'NONE',  ( 19.31922176934805435, 76.99660315353983719, -19.99999999999999645 ) ) ;
#21814=CARTESIAN_POINT ( 'NONE',  ( 41.00000000000000000, 103.4105893997321743, 27.49999999999999645 ) ) ;
#21823=CARTESIAN_POINT ( 'NONE',  ( -2.448772250512182280E-15, 99.94802294027086020, 27.49999999999999645 ) ) ;
#21831=AXIS2_PLACEMENT_3D ( 'NONE', #35861, #9777, #10175 ) ;
#21857=ORIENTED_EDGE ( 'NONE', *, *, #14837, .T. ) ;
#21860=VERTEX_POINT ( 'NONE', #3651 ) ;
#21866=ORIENTED_EDGE ( 'NONE', *, *, #11658, .T. ) ;
#21877=CARTESIAN_POINT ( 'NONE',  ( 0.000000000000000000, 101.4480229402710592, -24.99999999999999645 ) ) ;
#21880=ORIENTED_EDGE ( 'NONE', *, *, #31104, .T. ) ;
#21922=FACE_OUTER_BOUND ( 'NONE', #8461, .T. ) ;
#21940=VECTOR ( 'NONE', #34507, 1000.000000000000000 ) ;
#21961=DIRECTION ( 'NONE',  ( 0.000000000000000000, 0.000000000000000000, -1.000000000000000000 ) ) ;
#22020=ORIENTED_EDGE ( 'NONE', *, *, #21581, .F. ) ;
#22080=CARTESIAN_POINT ( 'NONE',  ( 37.50000000000000000, 103.4105893997321743, 18.49999999999999645 ) ) ;
#22114=CARTESIAN_POINT ( 'NONE',  ( 0.000000000000000000, 101.4480229402710734, 32.49999999999999289 ) ) ;
#22115=ORIENTED_EDGE ( 'NONE', *, *, #31811, .F. ) ;
#22118=AXIS2_PLACEMENT_3D ( 'NONE', #537, #4099, #11963 ) ;
#22127=CARTESIAN_POINT ( 'NONE',  ( 0.000000000000000000, 92.82302294027091705, 37.47964607176054130 ) ) ;
#22197=ORIENTED_EDGE ( 'NONE', *, *, #33351, .T. ) ;
#22247=VERTEX_POINT ( 'NONE', #21805 ) ;
#22320=ORIENTED_EDGE ( 'NONE', *, *, #34214, .F. ) ;
#22340=ORIENTED_EDGE ( 'NONE', *, *, #36814, .F. ) ;
#22342=PLANE ( 'NONE',  #4445 ) ;
#22358=EDGE_LOOP ( 'NONE', ( #283, #15161, #13875, #22775, #21724 ) ) ;
#22387=DIRECTION ( 'NONE',  ( 0.000000000000000000, 0.4999999999999951150, -0.8660254037844414832 ) ) ;
#22456=CIRCLE ( 'NONE', #5710, 8.500000000000003553 ) ;
#22470=AXIS2_PLACEMENT_3D ( 'NONE', #8128, #11485, #14112 ) ;
#22529=CARTESIAN_POINT ( 'NONE',  ( -5.750000000000000000, 89.94802294027094547, 32.49999999999999289 ) ) ;
#22542=DIRECTION ( 'NONE',  ( 1.000000000000000000, 0.000000000000000000, 0.000000000000000000 ) ) ;
#22558=DIRECTION ( 'NONE',  ( -1.000000000000000000, 0.000000000000000000, 0.000000000000000000 ) ) ;
#22559=FACE_OUTER_BOUND ( 'NONE', #32063, .T. ) ;
#22576=ORIENTED_EDGE ( 'NONE', *, *, #11240, .T. ) ;
#22591=CIRCLE ( 'NONE', #34564, 5.750000000000002665 ) ;
#22615=CIRCLE ( 'NONE', #34619, 8.500000000000000000 ) ;
#22680=FACE_BOUND ( 'NONE', #34979, .T. ) ;
#22733=ADVANCED_FACE ( 'NONE', ( #34829 ), #5970, .T. ) ;
#22739=DIRECTION ( 'NONE',  ( -0.000000000000000000, 0.000000000000000000, -1.000000000000000000 ) ) ;
#22748=EDGE_CURVE ( 'NONE', #6874, #16532, #35007, .T. ) ;
#22775=ORIENTED_EDGE ( 'NONE', *, *, #29029, .T. ) ;
#22793=ORIENTED_EDGE ( 'NONE', *, *, #26581, .F. ) ;
#22808=CARTESIAN_POINT ( 'NONE',  ( 33.99999999999999289, 103.4105893997321743, -19.99999999999999645 ) ) ;
#22822=CARTESIAN_POINT ( 'NONE',  ( 0.000000000000000000, 89.94802294027088863, -24.99999999999999645 ) ) ;
#22852=LINE ( 'NONE', #30907, #20867 ) ;
#22859=DIRECTION ( 'NONE',  ( 0.000000000000000000, 0.000000000000000000, -1.000000000000000000 ) ) ;
#22885=FACE_OUTER_BOUND ( 'NONE', #18543, .T. ) ;
#22898=CARTESIAN_POINT ( 'NONE',  ( 37.50000000000000000, 103.4105893997321743, 18.49999999999999645 ) ) ;
#22929=DIRECTION ( 'NONE',  ( -1.000000000000000000, 0.000000000000000000, 0.000000000000000000 ) ) ;
#22949=EDGE_CURVE ( 'NONE', #4610, #21860, #7624, .T. ) ;
#22966=EDGE_CURVE ( 'NONE', #20246, #25464, #8307, .T. ) ;
#22981=VECTOR ( 'NONE', #14093, 1000.000000000000114 ) ;
#23076=DIRECTION ( 'NONE',  ( 1.000000000000000000, 0.000000000000000000, 0.000000000000000000 ) ) ;
#23146=PRODUCT_DEFINITION_FORMATION_WITH_SPECIFIED_SOURCE ( 'ANY', '', #160, .NOT_KNOWN. ) ;
#23182=VECTOR ( 'NONE', #20070, 1000.000000000000000 ) ;
#23249=AXIS2_PLACEMENT_3D ( 'NONE', #4633, #16073, #19975 ) ;
#23252=DIRECTION ( 'NONE',  ( -1.000000000000000000, 0.000000000000000000, 0.000000000000000000 ) ) ;
#23270=DIRECTION ( 'NONE',  ( -0.7650473262243671080, -0.6439740589782688707, -0.000000000000000000 ) ) ;
#23271=VECTOR ( 'NONE', #27748, 1000.000000000000114 ) ;
#23306=DIRECTION ( 'NONE',  ( 0.000000000000000000, 0.4999999999999941713, -0.8660254037844420383 ) ) ;
#23398=CARTESIAN_POINT ( 'NONE',  ( 20.00000000000001066, 89.94802294027088863, 27.49999999999999645 ) ) ;
#23423=EDGE_CURVE ( 'NONE', #9029, #21384, #5245, .T. ) ;
#23424=DIRECTION ( 'NONE',  ( -0.000000000000000000, -0.000000000000000000, 1.000000000000000000 ) ) ;
#23435=ORIENTED_EDGE ( 'NONE', *, *, #14783, .F. ) ;
#23475=ORIENTED_EDGE ( 'NONE', *, *, #15491, .T. ) ;
#23497=ORIENTED_EDGE ( 'NONE', *, *, #681, .F. ) ;
#23505=EDGE_CURVE ( 'NONE', #4760, #105, #35202, .T. ) ;
#23514=ORIENTED_EDGE ( 'NONE', *, *, #31535, .T. ) ;
#23630=CARTESIAN_POINT ( 'NONE',  ( 19.53925848833874213, 89.94802294027088863, -23.27834620192013304 ) ) ;
#23717=EDGE_CURVE ( 'NONE', #26378, #27735, #17834, .T. ) ;
#23725=CIRCLE ( 'NONE', #11133, 100.0000000000000142 ) ;
#23732=CARTESIAN_POINT ( 'NONE',  ( -3.368272016354732390, 78.44802294027070388, -24.99999999999999645 ) ) ;
#23770=CARTESIAN_POINT ( 'NONE',  ( 2.143131898507887033E-16, 84.74289592134881843, -25.98445554337711627 ) ) ;
#23774=EDGE_CURVE ( 'NONE', #36432, #22247, #3970, .T. ) ;
#23777=FACE_OUTER_BOUND ( 'NONE', #24967, .T. ) ;
#23823=CARTESIAN_POINT ( 'NONE',  ( 3.368272016354729725, 78.44802294027070388, -24.99999999999999289 ) ) ;
#23828=ORIENTED_EDGE ( 'NONE', *, *, #469, .F. ) ;
#23899=DIRECTION ( 'NONE',  ( 0.000000000000000000, 0.000000000000000000, -1.000000000000000000 ) ) ;
#23912=EDGE_LOOP ( 'NONE', ( #31962, #8173 ) ) ;
#23950=FACE_OUTER_BOUND ( 'NONE', #26410, .T. ) ;
#24037=CARTESIAN_POINT ( 'NONE',  ( 40.98360655737705116, 111.1639425680974398, 27.49999999999999645 ) ) ;
#24069=ORIENTED_EDGE ( 'NONE', *, *, #31744, .F. ) ;
#24099=ORIENTED_EDGE ( 'NONE', *, *, #16710, .F. ) ;
#24118=ADVANCED_FACE ( 'NONE', ( #22885 ), #31682, .T. ) ;
#24132=AXIS2_PLACEMENT_3D ( 'NONE', #1579, #7223, #27255 ) ;
#24151=CIRCLE ( 'NONE', #4408, 30.00000000000001421 ) ;
#24206=CARTESIAN_POINT ( 'NONE',  ( 17.55872235085559652, 89.94802294027088863, -23.00000000000000000 ) ) ;
#24207=EDGE_CURVE ( 'NONE', #18201, #34855, #20859, .T. ) ;
#24242=CARTESIAN_POINT ( 'NONE',  ( -5.750000000000035527, 83.21147890756138565, 32.49999999999999289 ) ) ;
#24270=AXIS2_PLACEMENT_3D ( 'NONE', #27132, #7275, #26775 ) ;
#24283=DIRECTION ( 'NONE',  ( 1.000000000000000000, 0.000000000000000000, 0.000000000000000000 ) ) ;
#24289=LINE ( 'NONE', #13232, #20181 ) ;
#24294=AXIS2_PLACEMENT_3D ( 'NONE', #34562, #3779, #26471 ) ;
#24326=FACE_OUTER_BOUND ( 'NONE', #29065, .T. ) ;
#24328=CARTESIAN_POINT ( 'NONE',  ( 5.749999999999999112, 96.68456697298042002, -25.00000000000000000 ) ) ;
#24345=VERTEX_POINT ( 'NONE', #9112 ) ;
#24348=ORIENTED_EDGE ( 'NONE', *, *, #13572, .F. ) ;
#24360=AXIS2_PLACEMENT_3D ( 'NONE', #15696, #10429, #24520 ) ;
#24376=DIRECTION ( 'NONE',  ( -0.000000000000000000, -0.000000000000000000, 1.000000000000000000 ) ) ;
#24386=AXIS2_PLACEMENT_3D ( 'NONE', #11094, #25746, #22542 ) ;
#24398=FACE_OUTER_BOUND ( 'NONE', #36759, .T. ) ;
#24406=ORIENTED_EDGE ( 'NONE', *, *, #30490, .F. ) ;
#24410=EDGE_CURVE ( 'NONE', #3167, #6253, #36455, .T. ) ;
#24411=AXIS2_PLACEMENT_3D ( 'NONE', #11659, #2688, #36817 ) ;
#24419=PLANE ( 'NONE',  #21831 ) ;
#24423=DIRECTION ( 'NONE',  ( -0.000000000000000000, -0.8660254037844413721, -0.4999999999999952816 ) ) ;
#24464=CARTESIAN_POINT ( 'NONE',  ( 0.000000000000000000, 81.28776890242656350, -29.99999999999985434 ) ) ;
#24490=AXIS2_PLACEMENT_3D ( 'NONE', #162, #34493, #11784 ) ;
#24520=DIRECTION ( 'NONE',  ( 1.000000000000000000, 0.000000000000000000, 0.000000000000000000 ) ) ;
#24554=DIRECTION ( 'NONE',  ( 1.000000000000000000, 0.000000000000000000, -0.000000000000000000 ) ) ;
#24567=CARTESIAN_POINT ( 'NONE',  ( 5.749999999999999112, 96.68456697298042002, 32.49999999999999289 ) ) ;
#24571=DIRECTION ( 'NONE',  ( -0.000000000000000000, -0.000000000000000000, 1.000000000000000000 ) ) ;
#24577=LINE ( 'NONE', #36561, #5652 ) ;
#24607=DIRECTION ( 'NONE',  ( -0.000000000000000000, 0.000000000000000000, -1.000000000000000000 ) ) ;
#24613=CYLINDRICAL_SURFACE ( 'NONE', #11146, 30.00000000000001421 ) ;
#24658=CARTESIAN_POINT ( 'NONE',  ( 42.97377950131529190, 96.90768712682505281, -19.99999999999999645 ) ) ;
#24683=SHAPE_DEFINITION_REPRESENTATION ( #31296, #35880 ) ;
#24778=ADVANCED_FACE ( 'NONE', ( #30618 ), #31342, .T. ) ;
#24796=EDGE_CURVE ( 'NONE', #27057, #21230, #13136, .T. ) ;
#24827=CARTESIAN_POINT ( 'NONE',  ( -42.97377950131527058, 96.90768712682508124, -11.00000000000000000 ) ) ;
#24830=VECTOR ( 'NONE', #23424, 1000.000000000000000 ) ;
#24881=CIRCLE ( 'NONE', #29619, 8.500000000000007105 ) ;
#24906=ORIENTED_EDGE ( 'NONE', *, *, #33042, .F. ) ;
#24938=VERTEX_POINT ( 'NONE', #21156 ) ;
#24962=AXIS2_PLACEMENT_3D ( 'NONE', #6063, #32293, #20860 ) ;
#24967=EDGE_LOOP ( 'NONE', ( #29040, #21151, #6928, #21437 ) ) ;
#24985=VECTOR ( 'NONE', #7312, 1000.000000000000000 ) ;
#24989=FACE_OUTER_BOUND ( 'NONE', #18481, .T. ) ;
#25009=DIRECTION ( 'NONE',  ( -0.000000000000000000, -0.000000000000000000, 1.000000000000000000 ) ) ;
#25062=AXIS2_PLACEMENT_3D ( 'NONE', #31308, #5627, #17065 ) ;
#25075=LINE ( 'NONE', #28231, #25606 ) ;
#25078=AXIS2_PLACEMENT_3D ( 'NONE', #20103, #8855, #34362 ) ;
#25133=CARTESIAN_POINT ( 'NONE',  ( 0.000000000000000000, 89.94802294027094547, 32.49999999999999289 ) ) ;
#25142=DIRECTION ( 'NONE',  ( -0.000000000000000000, -0.000000000000000000, -1.000000000000000000 ) ) ;
#25188=ADVANCED_FACE ( 'NONE', ( #5218 ), #2582, .T. ) ;
#25193=ORIENTED_EDGE ( 'NONE', *, *, #2349, .T. ) ;
#25205=EDGE_CURVE ( 'NONE', #15973, #9156, #8954, .T. ) ;
#25262=CARTESIAN_POINT ( 'NONE',  ( -40.98360655737705827, 111.1639425680974398, -19.99999999999999645 ) ) ;
#25265=EDGE_CURVE ( 'NONE', #5579, #33065, #17952, .T. ) ;
#25289=AXIS2_PLACEMENT_3D ( 'NONE', #10172, #33203, #36042 ) ;
#25309=EDGE_LOOP ( 'NONE', ( #4164, #335, #9127, #36881 ) ) ;
#25321=EDGE_LOOP ( 'NONE', ( #4230, #21796, #15699, #17248 ) ) ;
#25357=FACE_OUTER_BOUND ( 'NONE', #26719, .T. ) ;
#25377=DIRECTION ( 'NONE',  ( 0.000000000000000000, -0.8660254037844420383, -0.4999999999999941713 ) ) ;
#25388=ORIENTED_EDGE ( 'NONE', *, *, #37064, .F. ) ;
#25397=ORIENTED_EDGE ( 'NONE', *, *, #4827, .T. ) ;
#25399=ORIENTED_EDGE ( 'NONE', *, *, #30097, .F. ) ;
#25422=ORIENTED_EDGE ( 'NONE', *, *, #10917, .T. ) ;
#25453=CARTESIAN_POINT ( 'NONE',  ( -17.55872235085560007, 89.94802294027088863, 30.49999999999999289 ) ) ;
#25460=VECTOR ( 'NONE', #15503, 1000.000000000000000 ) ;
#25463=ORIENTED_EDGE ( 'NONE', *, *, #469, .T. ) ;
#25464=VERTEX_POINT ( 'NONE', #4627 ) ;
#25495=( LENGTH_UNIT ( ) NAMED_UNIT ( * ) SI_UNIT ( .MILLI., .METRE. ) );
#25528=DIRECTION ( 'NONE',  ( -0.7650473262243671080, -0.6439740589782688707, -0.000000000000000000 ) ) ;
#25544=ORIENTED_EDGE ( 'NONE', *, *, #7196, .F. ) ;
#25563=DIRECTION ( 'NONE',  ( 0.000000000000000000, 0.000000000000000000, -1.000000000000000000 ) ) ;
#25606=VECTOR ( 'NONE', #13969, 1000.000000000000000 ) ;
#25721=ORIENTED_EDGE ( 'NONE', *, *, #15748, .F. ) ;
#25722=DIRECTION ( 'NONE',  ( -0.000000000000000000, -0.8660254037844414832, -0.4999999999999953371 ) ) ;
#25746=DIRECTION ( 'NONE',  ( 0.000000000000000000, 0.000000000000000000, 1.000000000000000000 ) ) ;
#25789=ORIENTED_EDGE ( 'NONE', *, *, #32835, .F. ) ;
#25799=CARTESIAN_POINT ( 'NONE',  ( 2.143131898507887033E-16, 80.41276890242660613, -28.48445554337708785 ) ) ;
#25856=DIRECTION ( 'NONE',  ( 0.000000000000000000, 0.000000000000000000, -1.000000000000000000 ) ) ;
#25862=ORIENTED_EDGE ( 'NONE', *, *, #7324, .F. ) ;
#25884=LINE ( 'NONE', #33973, #16397 ) ;
#26043=ORIENTED_EDGE ( 'NONE', *, *, #13572, .T. ) ;
#26127=ORIENTED_EDGE ( 'NONE', *, *, #12948, .F. ) ;
#26165=LINE ( 'NONE', #32144, #3956 ) ;
#26167=CIRCLE ( 'NONE', #3415, 2.000000000000000000 ) ;
#26199=CARTESIAN_POINT ( 'NONE',  ( -42.97377950131527058, 96.90768712682508124, 27.49999999999999645 ) ) ;
#26272=ORIENTED_EDGE ( 'NONE', *, *, #30255, .F. ) ;
#26368=ORIENTED_EDGE ( 'NONE', *, *, #12627, .F. ) ;
#26374=EDGE_CURVE ( 'NONE', #34855, #30183, #26167, .T. ) ;
#26378=VERTEX_POINT ( 'NONE', #24037 ) ;
#26396=ADVANCED_FACE ( 'NONE', ( #30022 ), #30196, .T. ) ;
#26410=EDGE_LOOP ( 'NONE', ( #19129, #17338, #12492, #32865 ) ) ;
#26425=CARTESIAN_POINT ( 'NONE',  ( 0.000000000000000000, 89.94802294027088863, -19.99999999999999645 ) ) ;
#26470=VERTEX_POINT ( 'NONE', #19880 ) ;
#26471=DIRECTION ( 'NONE',  ( -1.000000000000000000, 0.000000000000000000, 0.000000000000000000 ) ) ;
#26522=CARTESIAN_POINT ( 'NONE',  ( -37.50000000000000000, 103.4105893997321886, 27.49999999999999645 ) ) ;
#26544=AXIS2_PLACEMENT_3D ( 'NONE', #31994, #25856, #20767 ) ;
#26581=EDGE_CURVE ( 'NONE', #20688, #24345, #32611, .T. ) ;
#26592=DIRECTION ( 'NONE',  ( -0.000000000000000000, -0.000000000000000000, 1.000000000000000000 ) ) ;
#26619=EDGE_LOOP ( 'NONE', ( #31305, #35142, #7000 ) ) ;
#26706=DIRECTION ( 'NONE',  ( 0.000000000000000000, 0.000000000000000000, 1.000000000000000000 ) ) ;
#26710=DIRECTION ( 'NONE',  ( 1.000000000000000000, 0.000000000000000000, 0.000000000000000000 ) ) ;
#26719=EDGE_LOOP ( 'NONE', ( #29889, #12501, #34495, #18124 ) ) ;
#26746=LINE ( 'NONE', #10245, #25460 ) ;
#26762=CIRCLE ( 'NONE', #24360, 30.00000000000001421 ) ;
#26770=ORIENTED_EDGE ( 'NONE', *, *, #22748, .T. ) ;
#26775=DIRECTION ( 'NONE',  ( 1.000000000000000000, 0.000000000000000000, 0.000000000000000000 ) ) ;
#26779=AXIS2_PLACEMENT_3D ( 'NONE', #8328, #25563, #22558 ) ;
#26781=CARTESIAN_POINT ( 'NONE',  ( 0.000000000000000000, 89.94802294027094547, -24.99999999999999645 ) ) ;
#26878=ORIENTED_EDGE ( 'NONE', *, *, #4058, .T. ) ;
#26899=APPLICATION_CONTEXT ( 'automotive_design' ) ;
#26903=CIRCLE ( 'NONE', #16129, 8.500000000000003553 ) ;
#26960=PRESENTATION_STYLE_ASSIGNMENT (( #27518 ) ) ;
#26974=CARTESIAN_POINT ( 'NONE',  ( -40.98360655737705116, 111.1639425680974398, 18.49999999999999645 ) ) ;
#26992=( BOUNDED_CURVE ( )  B_SPLINE_CURVE ( 3, ( #22114, #10673, #24567, #19300 ),
 .UNSPECIFIED., .F., .F. ) 
 B_SPLINE_CURVE_WITH_KNOTS ( ( 4, 4 ),
 ( 3.141592653589793116, 4.712388980384689674 ),
 .UNSPECIFIED. ) 
 CURVE ( )  GEOMETRIC_REPRESENTATION_ITEM ( )  RATIONAL_B_SPLINE_CURVE ( ( 1.000000000000000000, 0.8047378541243649375, 0.8047378541243649375, 1.000000000000000000 ) ) 
 REPRESENTATION_ITEM ( '' )  );
#27013=ORIENTED_EDGE ( 'NONE', *, *, #24796, .F. ) ;
#27057=VERTEX_POINT ( 'NONE', #4025 ) ;
#27105=ADVANCED_FACE ( 'NONE', ( #32135, #34968 ), #34796, .T. ) ;
#27115=AXIS2_PLACEMENT_3D ( 'NONE', #26522, #4229, #9483 ) ;
#27132=CARTESIAN_POINT ( 'NONE',  ( 0.000000000000000000, 89.94802294027088863, 32.49999999999999289 ) ) ;
#27238=CIRCLE ( 'NONE', #2707, 5.750000000000002665 ) ;
#27255=DIRECTION ( 'NONE',  ( -0.7650473262243671080, -0.6439740589782688707, 0.000000000000000000 ) ) ;
#27321=EDGE_CURVE ( 'NONE', #6252, #35994, #33858, .T. ) ;
#27354=AXIS2_PLACEMENT_3D ( 'NONE', #17173, #28601, #3106 ) ;
#27386=CARTESIAN_POINT ( 'NONE',  ( 0.000000000000000000, 89.94802294027088863, 30.49999999999999289 ) ) ;
#27412=CARTESIAN_POINT ( 'NONE',  ( 0.000000000000000000, 101.4832769781154127, -24.97964607176053775 ) ) ;
#27426=ORIENTED_EDGE ( 'NONE', *, *, #23505, .F. ) ;
#27481=EDGE_CURVE ( 'NONE', #105, #4760, #14085, .T. ) ;
#27518=SURFACE_STYLE_USAGE ( .BOTH. , #10092 ) ;
#27560=DIRECTION ( 'NONE',  ( 0.000000000000000000, 0.000000000000000000, -1.000000000000000000 ) ) ;
#27595=DIRECTION ( 'NONE',  ( 1.000000000000000000, 0.000000000000000000, 0.000000000000000000 ) ) ;
#27696=ADVANCED_FACE ( 'NONE', ( #16172, #1907 ), #24419, .T. ) ;
#27720=CARTESIAN_POINT ( 'NONE',  ( -7.041719095097282852E-16, 78.41276890242659192, 32.52035392823930948 ) ) ;
#27735=VERTEX_POINT ( 'NONE', #31312 ) ;
#27743=AXIS2_PLACEMENT_3D ( 'NONE', #37027, #8882, #431 ) ;
#27748=DIRECTION ( 'NONE',  ( 0.000000000000000000, -0.8660254037844418162, 0.4999999999999945044 ) ) ;
#27840=ORIENTED_EDGE ( 'NONE', *, *, #12258, .T. ) ;
#27880=AXIS2_PLACEMENT_3D ( 'NONE', #9496, #29360, #24283 ) ;
#27964=AXIS2_PLACEMENT_3D ( 'NONE', #13598, #16603, #17152 ) ;
#27987=LINE ( 'NONE', #11470, #10082 ) ;
#27991=CARTESIAN_POINT ( 'NONE',  ( -37.50000000000000000, 103.4105893997321743, 18.49999999999999645 ) ) ;
#27993=ADVANCED_FACE ( 'NONE', ( #3743 ), #35272, .T. ) ;
#28092=AXIS2_PLACEMENT_3D ( 'NONE', #5665, #4934, #13749 ) ;
#28128=PRESENTATION_STYLE_ASSIGNMENT (( #3005 ) ) ;
#28173=CARTESIAN_POINT ( 'NONE',  ( 0.000000000000000000, 81.28776890242656350, 37.49999999999985079 ) ) ;
#28231=CARTESIAN_POINT ( 'NONE',  ( -19.31922176934808633, 76.99660315353983719, -19.99999999999999645 ) ) ;
#28243=CARTESIAN_POINT ( 'NONE',  ( -20.00000000000001066, 89.94802294027088863, 27.49999999999999645 ) ) ;
#28270=AXIS2_PLACEMENT_3D ( 'NONE', #11314, #2678, #34752 ) ;
#28332=PLANE ( 'NONE',  #36855 ) ;
#28337=VERTEX_POINT ( 'NONE', #12843 ) ;
#28340=CARTESIAN_POINT ( 'NONE',  ( -40.98360655737705827, 111.1639425680974398, 27.49999999999999645 ) ) ;
#28376=VERTEX_POINT ( 'NONE', #16059 ) ;
#28404=ORIENTED_EDGE ( 'NONE', *, *, #8071, .T. ) ;
#28409=AXIS2_PLACEMENT_3D ( 'NONE', #17452, #28512, #26 ) ;
#28469=DIRECTION ( 'NONE',  ( 0.000000000000000000, 0.4999999999999953926, 0.8660254037844412611 ) ) ;
#28505=DIRECTION ( 'NONE',  ( 0.000000000000000000, 0.000000000000000000, -1.000000000000000000 ) ) ;
#28512=DIRECTION ( 'NONE',  ( 0.000000000000000000, -0.8660254037844421493, -0.4999999999999942268 ) ) ;
#28520=CONICAL_SURFACE ( 'NONE', #983, 20.00000000000001066, 0.1396263401595466691 ) ;
#28524=FACE_OUTER_BOUND ( 'NONE', #8310, .T. ) ;
#28562=ORIENTED_EDGE ( 'NONE', *, *, #33351, .F. ) ;
#28601=DIRECTION ( 'NONE',  ( 0.000000000000000000, 0.000000000000000000, -1.000000000000000000 ) ) ;
#28632=CARTESIAN_POINT ( 'NONE',  ( -46.00000000000000000, 103.4105893997321886, 27.49999999999999645 ) ) ;
#28636=LINE ( 'NONE', #26199, #29909 ) ;
#28664=FACE_OUTER_BOUND ( 'NONE', #22358, .T. ) ;
#28668=UNCERTAINTY_MEASURE_WITH_UNIT (LENGTH_MEASURE( 1.000000000000000082E-05 ), #25495, 'distance_accuracy_value', 'NONE');
#28717=DIRECTION ( 'NONE',  ( -1.000000000000000000, 0.000000000000000000, 0.000000000000000000 ) ) ;
#28718=FACE_BOUND ( 'NONE', #3154, .T. ) ;
#28727=AXIS2_PLACEMENT_3D ( 'NONE', #9468, #24607, #651 ) ;
#28729=EDGE_CURVE ( 'NONE', #30923, #4610, #4585, .T. ) ;
#28731=VERTEX_POINT ( 'NONE', #21814 ) ;
#28764=VERTEX_POINT ( 'NONE', #1771 ) ;
#28773=EDGE_LOOP ( 'NONE', ( #6691, #9768, #36796, #31410 ) ) ;
#28841=DIRECTION ( 'NONE',  ( 0.000000000000000000, 0.000000000000000000, -1.000000000000000000 ) ) ;
#28970=ORIENTED_EDGE ( 'NONE', *, *, #30286, .T. ) ;
#29000=CARTESIAN_POINT ( 'NONE',  ( -37.50000000000000000, 103.4105893997321743, 18.49999999999999645 ) ) ;
#29029=EDGE_CURVE ( 'NONE', #15973, #28764, #20647, .T. ) ;
#29030=EDGE_LOOP ( 'NONE', ( #35618, #31709, #22320 ) ) ;
#29040=ORIENTED_EDGE ( 'NONE', *, *, #28729, .T. ) ;
#29065=EDGE_LOOP ( 'NONE', ( #23828, #9261, #35549, #19772 ) ) ;
#29078=VERTEX_POINT ( 'NONE', #13328 ) ;
#29097=COLOUR_RGB ( '', 0.31764706, 0.68627451, 0.89019608) ;
#29113=EDGE_LOOP ( 'NONE', ( #36299, #21400, #34388, #23435 ) ) ;
#29123=EDGE_CURVE ( 'NONE', #3432, #3167, #7526, .T. ) ;
#29156=AXIS2_PLACEMENT_3D ( 'NONE', #4343, #4530, #1513 ) ;
#29186=ADVANCED_FACE ( 'NONE', ( #15971 ), #24613, .T. ) ;
#29208=AXIS2_PLACEMENT_3D ( 'NONE', #3868, #17398, #6312 ) ;
#29284=DIRECTION ( 'NONE',  ( -0.000000000000000000, -0.000000000000000000, -1.000000000000000000 ) ) ;
#29286=CARTESIAN_POINT ( 'NONE',  ( 0.000000000000000000, 92.82302294027094547, 37.47964607176044183 ) ) ;
#29319=CARTESIAN_POINT ( 'NONE',  ( -17.55872235085559652, 89.94802294027088863, -23.00000000000000000 ) ) ;
#29341=CIRCLE ( 'NONE', #28727, 100.0000000000000142 ) ;
#29360=DIRECTION ( 'NONE',  ( -0.000000000000000000, -0.000000000000000000, 1.000000000000000000 ) ) ;
#29374=EDGE_CURVE ( 'NONE', #33050, #17955, #6179, .T. ) ;
#29383=AXIS2_PLACEMENT_3D ( 'NONE', #8586, #20560, #17022 ) ;
#29465=VERTEX_POINT ( 'NONE', #33162 ) ;
#29491=CARTESIAN_POINT ( 'NONE',  ( 37.50000000000000000, 103.4105893997321743, -19.99999999999999645 ) ) ;
#29497=ADVANCED_FACE ( 'NONE', ( #10126 ), #18980, .T. ) ;
#29519=EDGE_LOOP ( 'NONE', ( #11098, #17664, #31746, #4571, #25397 ) ) ;
#29551=CARTESIAN_POINT ( 'NONE',  ( 42.97377950131529190, 96.90768712682505281, -19.99999999999999645 ) ) ;
#29557=PLANE ( 'NONE',  #30557 ) ;
#29586=VECTOR ( 'NONE', #32219, 1000.000000000000000 ) ;
#29615=CARTESIAN_POINT ( 'NONE',  ( 0.000000000000000000, 101.4480229402710592, -24.99999999999999645 ) ) ;
#29619=AXIS2_PLACEMENT_3D ( 'NONE', #21444, #21799, #18453 ) ;
#29633=DIRECTION ( 'NONE',  ( -0.1391731009600657432, 0.000000000000000000, 0.9902680687415703620 ) ) ;
#29648=DIRECTION ( 'NONE',  ( 0.000000000000000000, -0.000000000000000000, 1.000000000000000000 ) ) ;
#29685=CARTESIAN_POINT ( 'NONE',  ( 28.99999999999998934, 103.4105893997321743, 18.49999999999999645 ) ) ;
#29708=DIRECTION ( 'NONE',  ( -1.000000000000000000, 0.000000000000000000, 0.000000000000000000 ) ) ;
#29714=FACE_OUTER_BOUND ( 'NONE', #7405, .T. ) ;
#29733=CARTESIAN_POINT ( 'NONE',  ( 42.97377950131527058, 96.90768712682506703, 18.49999999999999645 ) ) ;
#29775=( GEOMETRIC_REPRESENTATION_CONTEXT ( 3 ) GLOBAL_UNCERTAINTY_ASSIGNED_CONTEXT ( ( #34299 ) ) GLOBAL_UNIT_ASSIGNED_CONTEXT ( ( #8062, #14248, #14043 ) ) REPRESENTATION_CONTEXT ( 'NONE', 'WORKASPACE' ) );
#29878=DIRECTION ( 'NONE',  ( 1.000000000000000000, 0.000000000000000000, 0.000000000000000000 ) ) ;
#29889=ORIENTED_EDGE ( 'NONE', *, *, #20828, .F. ) ;
#29909=VECTOR ( 'NONE', #2967, 1000.000000000000000 ) ;
#29945=CARTESIAN_POINT ( 'NONE',  ( -41.00000000000000000, 103.4105893997321886, 27.49999999999999645 ) ) ;
#29953=CARTESIAN_POINT ( 'NONE',  ( 0.000000000000000000, 85.61789592134881843, -27.49999999999990408 ) ) ;
#29975=PLANE ( 'NONE',  #20888 ) ;
#29977=AXIS2_PLACEMENT_3D ( 'NONE', #5428, #27560, #33737 ) ;
#30018=EDGE_LOOP ( 'NONE', ( #11231, #33889, #3178, #20146, #8099 ) ) ;
#30022=FACE_OUTER_BOUND ( 'NONE', #33000, .T. ) ;
#30066=FACE_OUTER_BOUND ( 'NONE', #13530, .T. ) ;
#30081=ORIENTED_EDGE ( 'NONE', *, *, #1622, .T. ) ;
#30097=EDGE_CURVE ( 'NONE', #29465, #15238, #17322, .T. ) ;
#30146=EDGE_CURVE ( 'NONE', #28337, #16532, #4666, .T. ) ;
#30152=ORIENTED_EDGE ( 'NONE', *, *, #33143, .T. ) ;
#30183=VERTEX_POINT ( 'NONE', #11322 ) ;
#30196=CYLINDRICAL_SURFACE ( 'NONE', #29156, 5.750000000000002665 ) ;
#30204=AXIS2_PLACEMENT_3D ( 'NONE', #22898, #2478, #19536 ) ;
#30208=ORIENTED_EDGE ( 'NONE', *, *, #10977, .T. ) ;
#30210=CARTESIAN_POINT ( 'NONE',  ( -42.97377950131527058, 96.90768712682508124, 27.49999999999999645 ) ) ;
#30255=EDGE_CURVE ( 'NONE', #13946, #19982, #22615, .T. ) ;
#30286=EDGE_CURVE ( 'NONE', #4050, #28376, #32175, .T. ) ;
#30294=AXIS2_PLACEMENT_3D ( 'NONE', #4964, #20083, #33660 ) ;
#30326=ORIENTED_EDGE ( 'NONE', *, *, #33639, .T. ) ;
#30384=DIRECTION ( 'NONE',  ( 0.000000000000000000, 0.000000000000000000, 1.000000000000000000 ) ) ;
#30391=VECTOR ( 'NONE', #36870, 999.9999999999998863 ) ;
#30396=DIRECTION ( 'NONE',  ( -1.224646799147353207E-16, 1.000000000000000000, 0.000000000000000000 ) ) ;
#30417=AXIS2_PLACEMENT_3D ( 'NONE', #17640, #3411, #14847 ) ;
#30451=DIRECTION ( 'NONE',  ( -0.000000000000000000, -0.000000000000000000, -1.000000000000000000 ) ) ;
#30472=LINE ( 'NONE', #19591, #4153 ) ;
#30479=AXIS2_PLACEMENT_3D ( 'NONE', #3130, #6299, #34644 ) ;
#30490=EDGE_CURVE ( 'NONE', #8464, #28764, #6480, .T. ) ;
#30509=DIRECTION ( 'NONE',  ( 1.000000000000000000, 0.000000000000000000, 0.000000000000000000 ) ) ;
#30557=AXIS2_PLACEMENT_3D ( 'NONE', #18326, #3883, #14773 ) ;
#30560=CARTESIAN_POINT ( 'NONE',  ( -19.31922176934808633, 76.99660315353983719, -11.00000000000000000 ) ) ;
#30618=FACE_OUTER_BOUND ( 'NONE', #35943, .T. ) ;
#30622=ADVANCED_FACE ( 'NONE', ( #16729 ), #8824, .T. ) ;
#30645=CARTESIAN_POINT ( 'NONE',  ( -17.55872235085559652, 89.94802294027088863, -24.99999999999999645 ) ) ;
#30665=CARTESIAN_POINT ( 'NONE',  ( -20.00000000000001066, 89.94802294027088863, -19.99999999999999645 ) ) ;
#30682=CARTESIAN_POINT ( 'NONE',  ( 40.98360655737705116, 111.1639425680974398, -19.99999999999999645 ) ) ;
#30735=EDGE_LOOP ( 'NONE', ( #13519, #32831, #2228, #13818 ) ) ;
#30767=DIRECTION ( 'NONE',  ( 1.000000000000000000, 0.000000000000000000, 0.000000000000000000 ) ) ;
#30768=EDGE_LOOP ( 'NONE', ( #34132, #19152, #25193, #9538, #15356 ) ) ;
#30782=ORIENTED_EDGE ( 'NONE', *, *, #493, .F. ) ;
#30836=VERTEX_POINT ( 'NONE', #36373 ) ;
#30907=CARTESIAN_POINT ( 'NONE',  ( 33.99999999999999289, 103.4105893997321743, -19.99999999999999645 ) ) ;
#30923=VERTEX_POINT ( 'NONE', #30560 ) ;
#30948=EDGE_CURVE ( 'NONE', #6252, #530, #22852, .T. ) ;
#30967=CARTESIAN_POINT ( 'NONE',  ( 42.97377950131527058, 96.90768712682506703, 27.49999999999999645 ) ) ;
#30979=ORIENTED_EDGE ( 'NONE', *, *, #22949, .T. ) ;
#30982=ORIENTED_EDGE ( 'NONE', *, *, #30146, .T. ) ;
#31077=AXIS2_PLACEMENT_3D ( 'NONE', #26781, #1097, #12521 ) ;
#31104=EDGE_CURVE ( 'NONE', #33241, #27057, #6815, .T. ) ;
#31118=AXIS2_PLACEMENT_3D ( 'NONE', #5577, #17210, #8760 ) ;
#31153=CARTESIAN_POINT ( 'NONE',  ( 0.000000000000000000, 98.60827697811544112, -19.99999999999999645 ) ) ;
#31161=AXIS2_PLACEMENT_3D ( 'NONE', #5832, #11609, #9370 ) ;
#31168=DIRECTION ( 'NONE',  ( -0.000000000000000000, -0.000000000000000000, 1.000000000000000000 ) ) ;
#31197=CARTESIAN_POINT ( 'NONE',  ( -42.97377950131527058, 96.90768712682508124, 18.49999999999999645 ) ) ;
#31213=ORIENTED_EDGE ( 'NONE', *, *, #10802, .F. ) ;
#31239=DIRECTION ( 'NONE',  ( -0.000000000000000000, -0.000000000000000000, 1.000000000000000000 ) ) ;
#31241=DIRECTION ( 'NONE',  ( 0.000000000000000000, 0.000000000000000000, -1.000000000000000000 ) ) ;
#31282=CARTESIAN_POINT ( 'NONE',  ( 0.000000000000000000, 89.94802294027097389, 32.49999999999990052 ) ) ;
#31289=CIRCLE ( 'NONE', #12704, 8.500000000000000000 ) ;
#31294=SURFACE_STYLE_FILL_AREA ( #5266 ) ;
#31296=PRODUCT_DEFINITION_SHAPE ( 'NONE', 'NONE',  #15978 ) ;
#31297=DIRECTION ( 'NONE',  ( -0.000000000000000000, -0.8660254037844420383, -0.4999999999999941713 ) ) ;
#31303=EDGE_LOOP ( 'NONE', ( #28970, #30326, #3796, #441, #35431, #22020, #34409, #6236 ) ) ;
#31305=ORIENTED_EDGE ( 'NONE', *, *, #19330, .F. ) ;
#31308=CARTESIAN_POINT ( 'NONE',  ( 0.000000000000000000, 89.94802294027097389, -24.99999999999990763 ) ) ;
#31312=CARTESIAN_POINT ( 'NONE',  ( 46.00000000000000000, 103.4105893997321743, 27.49999999999999645 ) ) ;
#31342=PLANE ( 'NONE',  #28092 ) ;
#31381=FACE_OUTER_BOUND ( 'NONE', #10745, .T. ) ;
#31410=ORIENTED_EDGE ( 'NONE', *, *, #17199, .F. ) ;
#31417=EDGE_CURVE ( 'NONE', #13656, #12615, #6841, .T. ) ;
#31456=ORIENTED_EDGE ( 'NONE', *, *, #21287, .F. ) ;
#31457=( GEOMETRIC_REPRESENTATION_CONTEXT ( 3 ) GLOBAL_UNCERTAINTY_ASSIGNED_CONTEXT ( ( #9941 ) ) GLOBAL_UNIT_ASSIGNED_CONTEXT ( ( #37074, #8005, #14183 ) ) REPRESENTATION_CONTEXT ( 'NONE', 'WORKASPACE' ) );
#31468=LINE ( 'NONE', #544, #24830 ) ;
#31526=CYLINDRICAL_SURFACE ( 'NONE', #11179, 1.750000000000015765 ) ;
#31535=EDGE_CURVE ( 'NONE', #3432, #26470, #9236, .T. ) ;
#31542=AXIS2_PLACEMENT_3D ( 'NONE', #36523, #4450, #7837 ) ;
#31604=CARTESIAN_POINT ( 'NONE',  ( 7.041719095097282852E-16, 78.44802294027068967, -24.99999999999999645 ) ) ;
#31672=EDGE_CURVE ( 'NONE', #28731, #530, #18211, .T. ) ;
#31679=DIRECTION ( 'NONE',  ( 0.000000000000000000, 0.000000000000000000, -1.000000000000000000 ) ) ;
#31680=ADVANCED_FACE ( 'NONE', ( #24989 ), #22342, .F. ) ;
#31682=CYLINDRICAL_SURFACE ( 'NONE', #25062, 5.750000000000005329 ) ;
#31705=CARTESIAN_POINT ( 'NONE',  ( -2.775557561562891351E-14, 19.94802294027085310, -19.99999999999999645 ) ) ;
#31709=ORIENTED_EDGE ( 'NONE', *, *, #19330, .T. ) ;
#31733=CARTESIAN_POINT ( 'NONE',  ( -17.55872235085560007, 89.94802294027088863, 32.49999999999999289 ) ) ;
#31742=CARTESIAN_POINT ( 'NONE',  ( 0.000000000000000000, 101.4480229402710734, 32.49999999999999289 ) ) ;
#31744=EDGE_CURVE ( 'NONE', #12615, #17955, #32614, .T. ) ;
#31746=ORIENTED_EDGE ( 'NONE', *, *, #36476, .F. ) ;
#31781=TOROIDAL_SURFACE ( 'NONE', #29383, 17.55872235085559652, 2.000000000000000000 ) ;
#31800=FACE_OUTER_BOUND ( 'NONE', #31818, .T. ) ;
#31811=EDGE_CURVE ( 'NONE', #25464, #20246, #1488, .T. ) ;
#31818=EDGE_LOOP ( 'NONE', ( #11634, #23514, #10891, #32249, #5329 ) ) ;
#31839=CARTESIAN_POINT ( 'NONE',  ( 19.53925848833874213, 89.94802294027088863, 30.77834620192012594 ) ) ;
#31855=EDGE_CURVE ( 'NONE', #33050, #20027, #14826, .T. ) ;
#31895=CARTESIAN_POINT ( 'NONE',  ( -37.50000000000000000, 103.4105893997321886, -19.99999999999999645 ) ) ;
#31933=EDGE_CURVE ( 'NONE', #9156, #4556, #10687, .T. ) ;
#31958=VECTOR ( 'NONE', #31297, 1000.000000000000114 ) ;
#31962=ORIENTED_EDGE ( 'NONE', *, *, #681, .T. ) ;
#31981=CIRCLE ( 'NONE', #15255, 3.500000000000003109 ) ;
#31994=CARTESIAN_POINT ( 'NONE',  ( -2.448772250512182280E-15, 99.94802294027086020, 27.49999999999999645 ) ) ;
#31997=EDGE_LOOP ( 'NONE', ( #4922, #25463, #13491, #25862 ) ) ;
#32026=AXIS2_PLACEMENT_3D ( 'NONE', #11629, #31168, #5853 ) ;
#32063=EDGE_LOOP ( 'NONE', ( #134, #23475 ) ) ;
#32113=DIRECTION ( 'NONE',  ( -0.000000000000000000, -1.000000000000000000, -0.000000000000000000 ) ) ;
#32130=ORIENTED_EDGE ( 'NONE', *, *, #31855, .T. ) ;
#32135=FACE_OUTER_BOUND ( 'NONE', #14804, .T. ) ;
#32138=DIRECTION ( 'NONE',  ( -0.000000000000000000, -0.000000000000000000, 1.000000000000000000 ) ) ;
#32139=ADVANCED_FACE ( 'NONE', ( #36921, #2437, #22680 ), #20230, .F. ) ;
#32141=FACE_OUTER_BOUND ( 'NONE', #31303, .T. ) ;
#32144=CARTESIAN_POINT ( 'NONE',  ( -19.31922176934808633, 76.99660315353983719, 27.49999999999999645 ) ) ;
#32146=CIRCLE ( 'NONE', #11196, 17.55872235085559652 ) ;
#32158=CYLINDRICAL_SURFACE ( 'NONE', #27880, 8.500000000000003553 ) ;
#32175=CIRCLE ( 'NONE', #32811, 8.500000000000007105 ) ;
#32219=DIRECTION ( 'NONE',  ( 0.000000000000000000, 0.000000000000000000, -1.000000000000000000 ) ) ;
#32249=ORIENTED_EDGE ( 'NONE', *, *, #12582, .T. ) ;
#32292=DIRECTION ( 'NONE',  ( 0.000000000000000000, 0.000000000000000000, -1.000000000000000000 ) ) ;
#32293=DIRECTION ( 'NONE',  ( -0.000000000000000000, -0.000000000000000000, -1.000000000000000000 ) ) ;
#32325=FACE_OUTER_BOUND ( 'NONE', #30768, .T. ) ;
#32339=CARTESIAN_POINT ( 'NONE',  ( 5.750000000000000000, 89.94802294027094547, -24.99999999999999645 ) ) ;
#32342=ORIENTED_EDGE ( 'NONE', *, *, #13926, .T. ) ;
#32433=CARTESIAN_POINT ( 'NONE',  ( 28.99999999999999289, 103.4105893997321743, -19.99999999999999645 ) ) ;
#32479=EDGE_LOOP ( 'NONE', ( #35990, #25422, #25789, #31213, #2814, #26043, #18560, #24069 ) ) ;
#32508=MANIFOLD_SOLID_BREP ( 'Fillet1', #34554 ) ;
#32532=CIRCLE ( 'NONE', #27743, 17.55872235085560007 ) ;
#32566=DIRECTION ( 'NONE',  ( 1.000000000000000000, 0.000000000000000000, 0.000000000000000000 ) ) ;
#32611=CIRCLE ( 'NONE', #8049, 20.00000000000001066 ) ;
#32614=CIRCLE ( 'NONE', #30204, 8.500000000000007105 ) ;
#32666=CIRCLE ( 'NONE', #32026, 19.53925848833874213 ) ;
#32678=CARTESIAN_POINT ( 'NONE',  ( -7.041719095097282852E-16, 78.44802294027068967, 32.49999999999999289 ) ) ;
#32690=ORIENTED_EDGE ( 'NONE', *, *, #27321, .F. ) ;
#32739=EDGE_CURVE ( 'NONE', #29078, #30836, #26165, .T. ) ;
#32811=AXIS2_PLACEMENT_3D ( 'NONE', #3978, #29648, #21217 ) ;
#32831=ORIENTED_EDGE ( 'NONE', *, *, #19407, .F. ) ;
#32835=EDGE_CURVE ( 'NONE', #36432, #29465, #36275, .T. ) ;
#32865=ORIENTED_EDGE ( 'NONE', *, *, #31811, .T. ) ;
#32876=CIRCLE ( 'NONE', #31077, 5.750000000000005329 ) ;
#32877=ORIENTED_EDGE ( 'NONE', *, *, #22966, .F. ) ;
#32884=DIRECTION ( 'NONE',  ( -0.000000000000000000, -0.000000000000000000, 1.000000000000000000 ) ) ;
#32903=PLANE ( 'NONE',  #24132 ) ;
#32918=AXIS2_PLACEMENT_3D ( 'NONE', #25453, #11201, #11555 ) ;
#32968=CARTESIAN_POINT ( 'NONE',  ( -42.97377950131527058, 96.90768712682508124, 27.49999999999999645 ) ) ;
#32984=ORIENTED_EDGE ( 'NONE', *, *, #11463, .T. ) ;
#32991=DIRECTION ( 'NONE',  ( -1.000000000000000000, 0.000000000000000000, 0.000000000000000000 ) ) ;
#33000=EDGE_LOOP ( 'NONE', ( #33788, #26127, #35617 ) ) ;
#33037=DIRECTION ( 'NONE',  ( 0.6439740589782694258, 0.7650473262243666639, 0.000000000000000000 ) ) ;
#33038=EDGE_CURVE ( 'NONE', #30836, #33241, #2516, .T. ) ;
#33042=EDGE_CURVE ( 'NONE', #29078, #9029, #3242, .T. ) ;
#33050=VERTEX_POINT ( 'NONE', #14666 ) ;
#33052=EDGE_LOOP ( 'NONE', ( #36789, #1872 ) ) ;
#33065=VERTEX_POINT ( 'NONE', #31733 ) ;
#33104=DIRECTION ( 'NONE',  ( 0.000000000000000000, 0.4999999999999959477, -0.8660254037844409281 ) ) ;
#33123=FACE_OUTER_BOUND ( 'NONE', #36112, .T. ) ;
#33143=EDGE_CURVE ( 'NONE', #10852, #30836, #21354, .T. ) ;
#33162=CARTESIAN_POINT ( 'NONE',  ( 42.97377950131529190, 96.90768712682505281, -11.00000000000000000 ) ) ;
#33203=DIRECTION ( 'NONE',  ( -0.000000000000000000, -0.000000000000000000, 1.000000000000000000 ) ) ;
#33204=CARTESIAN_POINT ( 'NONE',  ( -2.448772250512182280E-15, 99.94802294027086020, -19.99999999999999645 ) ) ;
#33241=VERTEX_POINT ( 'NONE', #3980 ) ;
#33254=ADVANCED_FACE ( 'NONE', ( #35868 ), #12769, .F. ) ;
#33261=DIRECTION ( 'NONE',  ( -0.000000000000000000, -0.000000000000000000, -1.000000000000000000 ) ) ;
#33281=DIRECTION ( 'NONE',  ( 0.000000000000000000, 0.000000000000000000, -1.000000000000000000 ) ) ;
#33315=DIRECTION ( 'NONE',  ( -0.000000000000000000, -0.000000000000000000, -1.000000000000000000 ) ) ;
#33339=CARTESIAN_POINT ( 'NONE',  ( 5.750000000000000000, 89.94802294027094547, 32.49999999999999289 ) ) ;
#33351=EDGE_CURVE ( 'NONE', #21860, #36148, #9979, .T. ) ;
#33361=ORIENTED_EDGE ( 'NONE', *, *, #4596, .F. ) ;
#33374=DIRECTION ( 'NONE',  ( 1.000000000000000000, 0.000000000000000000, 0.000000000000000000 ) ) ;
#33383=CIRCLE ( 'NONE', #2222, 2.000000000000001776 ) ;
#33409=ORIENTED_EDGE ( 'NONE', *, *, #36476, .T. ) ;
#33412=CIRCLE ( 'NONE', #13652, 5.750000000000002665 ) ;
#33498=CIRCLE ( 'NONE', #22118, 8.500000000000000000 ) ;
#33576=EDGE_CURVE ( 'NONE', #755, #36148, #8633, .T. ) ;
#33589=DIRECTION ( 'NONE',  ( 0.000000000000000000, 0.000000000000000000, -1.000000000000000000 ) ) ;
#33639=EDGE_CURVE ( 'NONE', #28376, #12615, #1690, .T. ) ;
#33660=DIRECTION ( 'NONE',  ( -1.000000000000000000, 0.000000000000000000, 0.000000000000000000 ) ) ;
#33716=AXIS2_PLACEMENT_3D ( 'NONE', #6481, #18475, #26710 ) ;
#33737=DIRECTION ( 'NONE',  ( -1.000000000000000000, 0.000000000000000000, 0.000000000000000000 ) ) ;
#33752=ORIENTED_EDGE ( 'NONE', *, *, #30146, .F. ) ;
#33762=EDGE_CURVE ( 'NONE', #3254, #15973, #22591, .T. ) ;
#33788=ORIENTED_EDGE ( 'NONE', *, *, #11493, .F. ) ;
#33789=ORIENTED_EDGE ( 'NONE', *, *, #13494, .F. ) ;
#33796=ORIENTED_EDGE ( 'NONE', *, *, #31672, .F. ) ;
#33858=CIRCLE ( 'NONE', #22470, 3.500000000000003109 ) ;
#33889=ORIENTED_EDGE ( 'NONE', *, *, #1622, .F. ) ;
#33952=LINE ( 'NONE', #2454, #23271 ) ;
#33973=CARTESIAN_POINT ( 'NONE',  ( -40.98360655737705827, 111.1639425680974398, 27.49999999999999645 ) ) ;
#33990=TOROIDAL_SURFACE ( 'NONE', #10022, 17.55872235085560007, 2.000000000000000000 ) ;
#34132=ORIENTED_EDGE ( 'NONE', *, *, #22748, .F. ) ;
#34169=DIRECTION ( 'NONE',  ( 0.000000000000000000, -0.000000000000000000, 1.000000000000000000 ) ) ;
#34214=EDGE_CURVE ( 'NONE', #26470, #6533, #5782, .T. ) ;
#34299=UNCERTAINTY_MEASURE_WITH_UNIT (LENGTH_MEASURE( 1.000000000000000082E-05 ), #8062, 'distance_accuracy_value', 'NONE');
#34362=DIRECTION ( 'NONE',  ( -1.000000000000000000, 0.000000000000000000, 0.000000000000000000 ) ) ;
#34388=ORIENTED_EDGE ( 'NONE', *, *, #37064, .T. ) ;
#34409=ORIENTED_EDGE ( 'NONE', *, *, #35963, .F. ) ;
#34484=DIRECTION ( 'NONE',  ( 0.000000000000000000, 0.000000000000000000, -1.000000000000000000 ) ) ;
#34491=CARTESIAN_POINT ( 'NONE',  ( 37.50000000000000000, 103.4105893997321743, -19.99999999999999645 ) ) ;
#34492=VECTOR ( 'NONE', #13011, 1000.000000000000000 ) ;
#34493=DIRECTION ( 'NONE',  ( -0.000000000000000000, 0.000000000000000000, -1.000000000000000000 ) ) ;
#34495=ORIENTED_EDGE ( 'NONE', *, *, #2945, .F. ) ;
#34506=DIRECTION ( 'NONE',  ( 0.000000000000000000, 0.000000000000000000, -1.000000000000000000 ) ) ;
#34507=DIRECTION ( 'NONE',  ( 0.000000000000000000, 0.000000000000000000, -1.000000000000000000 ) ) ;
#34554=CLOSED_SHELL ( 'NONE', ( #16534, #8, #27993, #36919, #8402, #5448, #24118, #22733, #29497, #2092, #12707, #25188, #18799, #16064, #4626, #11734, #10936, #18002, #18763, #29186, #12765, #35877, #2207, #21802, #18108, #27696, #5904, #30622, #6576, #21583, #17876, #32139, #13297, #31680, #35336, #33254, #5181, #27105, #24778, #26396, #3819, #10065, #8514 ) ) ;
#34559=PLANE ( 'NONE',  #34863 ) ;
#34562=CARTESIAN_POINT ( 'NONE',  ( -37.50000000000000000, 103.4105893997321886, -19.99999999999999645 ) ) ;
#34564=AXIS2_PLACEMENT_3D ( 'NONE', #25133, #7877, #14027 ) ;
#34619=AXIS2_PLACEMENT_3D ( 'NONE', #31895, #32292, #3785 ) ;
#34644=DIRECTION ( 'NONE',  ( 0.000000000000000000, 0.4999999999999953926, -0.8660254037844412611 ) ) ;
#34677=CARTESIAN_POINT ( 'NONE',  ( -33.99999999999999289, 103.4105893997321886, 27.49999999999999645 ) ) ;
#34697=ORIENTED_EDGE ( 'NONE', *, *, #36814, .T. ) ;
#34752=DIRECTION ( 'NONE',  ( -1.000000000000000000, 0.000000000000000000, 0.000000000000000000 ) ) ;
#34796=PLANE ( 'NONE',  #18873 ) ;
#34829=FACE_OUTER_BOUND ( 'NONE', #29030, .T. ) ;
#34838=DIRECTION ( 'NONE',  ( -0.000000000000000000, -0.000000000000000000, 1.000000000000000000 ) ) ;
#34848=FACE_OUTER_BOUND ( 'NONE', #30018, .T. ) ;
#34855=VERTEX_POINT ( 'NONE', #23630 ) ;
#34863=AXIS2_PLACEMENT_3D ( 'NONE', #8862, #25377, #23306 ) ;
#34875=ORIENTED_EDGE ( 'NONE', *, *, #31744, .T. ) ;
#34881=( BOUNDED_CURVE ( )  B_SPLINE_CURVE ( 3, ( #32678, #12789, #24242, #10199 ),
 .UNSPECIFIED., .F., .F. ) 
 B_SPLINE_CURVE_WITH_KNOTS ( ( 4, 4 ),
 ( 1.224646799147352468E-16, 1.570796326794907438 ),
 .UNSPECIFIED. ) 
 CURVE ( )  GEOMETRIC_REPRESENTATION_ITEM ( )  RATIONAL_B_SPLINE_CURVE ( ( 1.000000000000000000, 0.8047378541243626060, 0.8047378541243626060, 1.000000000000000000 ) ) 
 REPRESENTATION_ITEM ( '' )  );
#34894=CARTESIAN_POINT ( 'NONE',  ( 7.041719095097282852E-16, 78.44802294027068967, -24.99999999999999645 ) ) ;
#34912=DIRECTION ( 'NONE',  ( 0.000000000000000000, 0.4999999999999959477, -0.8660254037844409281 ) ) ;
#34952=DIRECTION ( 'NONE',  ( -1.000000000000000000, 0.000000000000000000, 0.000000000000000000 ) ) ;
#34968=FACE_BOUND ( 'NONE', #5941, .T. ) ;
#34979=EDGE_LOOP ( 'NONE', ( #15747, #10035 ) ) ;
#35007=LINE ( 'NONE', #23398, #5892 ) ;
#35081=CARTESIAN_POINT ( 'NONE',  ( -33.99999999999999289, 103.4105893997321886, -19.99999999999999645 ) ) ;
#35142=ORIENTED_EDGE ( 'NONE', *, *, #554, .T. ) ;
#35202=CIRCLE ( 'NONE', #26779, 3.500000000000003109 ) ;
#35221=ORIENTED_EDGE ( 'NONE', *, *, #35492, .F. ) ;
#35251=CARTESIAN_POINT ( 'NONE',  ( -42.97377950131527058, 96.90768712682508124, -19.99999999999999645 ) ) ;
#35272=CYLINDRICAL_SURFACE ( 'NONE', #8077, 5.750000000000002665 ) ;
#35275=CARTESIAN_POINT ( 'NONE',  ( 7.041719095097282852E-16, 78.44802294027068967, -24.99999999999999645 ) ) ;
#35321=DIRECTION ( 'NONE',  ( -0.7650473262243665529, 0.6439740589782693148, 0.000000000000000000 ) ) ;
#35336=ADVANCED_FACE ( 'NONE', ( #34848 ), #9142, .T. ) ;
#35367=PLANE ( 'NONE',  #2405 ) ;
#35431=ORIENTED_EDGE ( 'NONE', *, *, #23717, .T. ) ;
#35456=EDGE_LOOP ( 'NONE', ( #11834, #14539, #17579, #15373, #24099 ) ) ;
#35492=EDGE_CURVE ( 'NONE', #33065, #374, #3895, .T. ) ;
#35525=ORIENTED_EDGE ( 'NONE', *, *, #2349, .F. ) ;
#35527=CARTESIAN_POINT ( 'NONE',  ( 0.000000000000000000, 92.82302294027091705, -29.97964607176054130 ) ) ;
#35549=ORIENTED_EDGE ( 'NONE', *, *, #7324, .T. ) ;
#35579=ORIENTED_EDGE ( 'NONE', *, *, #10917, .F. ) ;
#35593=AXIS2_PLACEMENT_3D ( 'NONE', #2620, #33589, #2262 ) ;
#35617=ORIENTED_EDGE ( 'NONE', *, *, #33762, .T. ) ;
#35618=ORIENTED_EDGE ( 'NONE', *, *, #13494, .T. ) ;
#35861=CARTESIAN_POINT ( 'NONE',  ( 0.000000000000000000, 89.94802294027088863, -24.99999999999999645 ) ) ;
#35863=CIRCLE ( 'NONE', #24490, 30.00000000000001421 ) ;
#35866=DIRECTION ( 'NONE',  ( -0.000000000000000000, 0.8660254037844420383, -0.4999999999999945599 ) ) ;
#35868=FACE_OUTER_BOUND ( 'NONE', #8288, .T. ) ;
#35877=ADVANCED_FACE ( 'NONE', ( #29714 ), #32158, .T. ) ;
#35880=SHAPE_REPRESENTATION ( 'Pneumatic caliper', ( #21385 ), #29775 ) ;
#35917=DIRECTION ( 'NONE',  ( -0.000000000000000000, -0.000000000000000000, 1.000000000000000000 ) ) ;
#35943=EDGE_LOOP ( 'NONE', ( #17244, #24406 ) ) ;
#35957=EDGE_CURVE ( 'NONE', #19694, #28337, #36884, .T. ) ;
#35963=EDGE_CURVE ( 'NONE', #623, #8343, #5755, .T. ) ;
#35974=ORIENTED_EDGE ( 'NONE', *, *, #19018, .F. ) ;
#35990=ORIENTED_EDGE ( 'NONE', *, *, #33639, .F. ) ;
#35994=VERTEX_POINT ( 'NONE', #5852 ) ;
#36042=DIRECTION ( 'NONE',  ( -1.000000000000000000, 0.000000000000000000, 0.000000000000000000 ) ) ;
#36112=EDGE_LOOP ( 'NONE', ( #19529, #13140, #33796, #9334 ) ) ;
#36148=VERTEX_POINT ( 'NONE', #20279 ) ;
#36272=VERTEX_POINT ( 'NONE', #23770 ) ;
#36275=LINE ( 'NONE', #24658, #958 ) ;
#36288=CARTESIAN_POINT ( 'NONE',  ( 37.50000000000000000, 103.4105893997321743, -19.99999999999999645 ) ) ;
#36299=ORIENTED_EDGE ( 'NONE', *, *, #26374, .F. ) ;
#36324=VECTOR ( 'NONE', #21770, 1000.000000000000114 ) ;
#36334=AXIS2_PLACEMENT_3D ( 'NONE', #8091, #34169, #30767 ) ;
#36373=CARTESIAN_POINT ( 'NONE',  ( -19.31922176934808633, 76.99660315353983719, 18.49999999999999645 ) ) ;
#36384=CARTESIAN_POINT ( 'NONE',  ( 37.50000000000000000, 103.4105893997321743, 27.49999999999999645 ) ) ;
#36396=DIRECTION ( 'NONE',  ( 1.000000000000000000, 0.000000000000000000, 0.000000000000000000 ) ) ;
#36432=VERTEX_POINT ( 'NONE', #29551 ) ;
#36455=CIRCLE ( 'NONE', #30479, 5.750000000000002665 ) ;
#36472=VERTEX_POINT ( 'NONE', #29945 ) ;
#36476=EDGE_CURVE ( 'NONE', #24345, #16958, #26762, .T. ) ;
#36523=CARTESIAN_POINT ( 'NONE',  ( -2.448772250512182280E-15, 99.94802294027086020, 27.49999999999999645 ) ) ;
#36561=CARTESIAN_POINT ( 'NONE',  ( 41.00000000000000000, 103.4105893997321743, -19.99999999999999645 ) ) ;
#36583=DIRECTION ( 'NONE',  ( -0.000000000000000000, -0.000000000000000000, 1.000000000000000000 ) ) ;
#36736=ORIENTED_EDGE ( 'NONE', *, *, #30490, .T. ) ;
#36759=EDGE_LOOP ( 'NONE', ( #15916, #14622, #22576, #35221 ) ) ;
#36789=ORIENTED_EDGE ( 'NONE', *, *, #2294, .T. ) ;
#36796=ORIENTED_EDGE ( 'NONE', *, *, #19829, .T. ) ;
#36814=EDGE_CURVE ( 'NONE', #19982, #21384, #24289, .T. ) ;
#36817=DIRECTION ( 'NONE',  ( -1.000000000000000000, 0.000000000000000000, 0.000000000000000000 ) ) ;
#36818=DIRECTION ( 'NONE',  ( -0.7650473262243666639, 0.6439740589782693148, 0.000000000000000000 ) ) ;
#36855=AXIS2_PLACEMENT_3D ( 'NONE', #31705, #585, #17090 ) ;
#36870=DIRECTION ( 'NONE',  ( -0.1391731009600657432, 0.000000000000000000, -0.9902680687415703620 ) ) ;
#36871=DIRECTION ( 'NONE',  ( -1.000000000000000000, 0.000000000000000000, 0.000000000000000000 ) ) ;
#36881=ORIENTED_EDGE ( 'NONE', *, *, #20477, .F. ) ;
#36884=CIRCLE ( 'NONE', #30294, 20.00000000000001066 ) ;
#36919=ADVANCED_FACE ( 'NONE', ( #31381 ), #5712, .T. ) ;
#36921=FACE_OUTER_BOUND ( 'NONE', #11808, .T. ) ;
#36939=SURFACE_SIDE_STYLE ('',( #31294 ) ) ;
#36950=ORIENTED_EDGE ( 'NONE', *, *, #25205, .T. ) ;
#36979=CYLINDRICAL_SURFACE ( 'NONE', #11296, 100.0000000000000142 ) ;
#37027=CARTESIAN_POINT ( 'NONE',  ( 0.000000000000000000, 89.94802294027088863, 32.49999999999999289 ) ) ;
#37064=EDGE_CURVE ( 'NONE', #18201, #4131, #33383, .T. ) ;
#37074=( LENGTH_UNIT ( ) NAMED_UNIT ( * ) SI_UNIT ( .MILLI., .METRE. ) );
ENDSEC;
END-ISO-10303-21;
